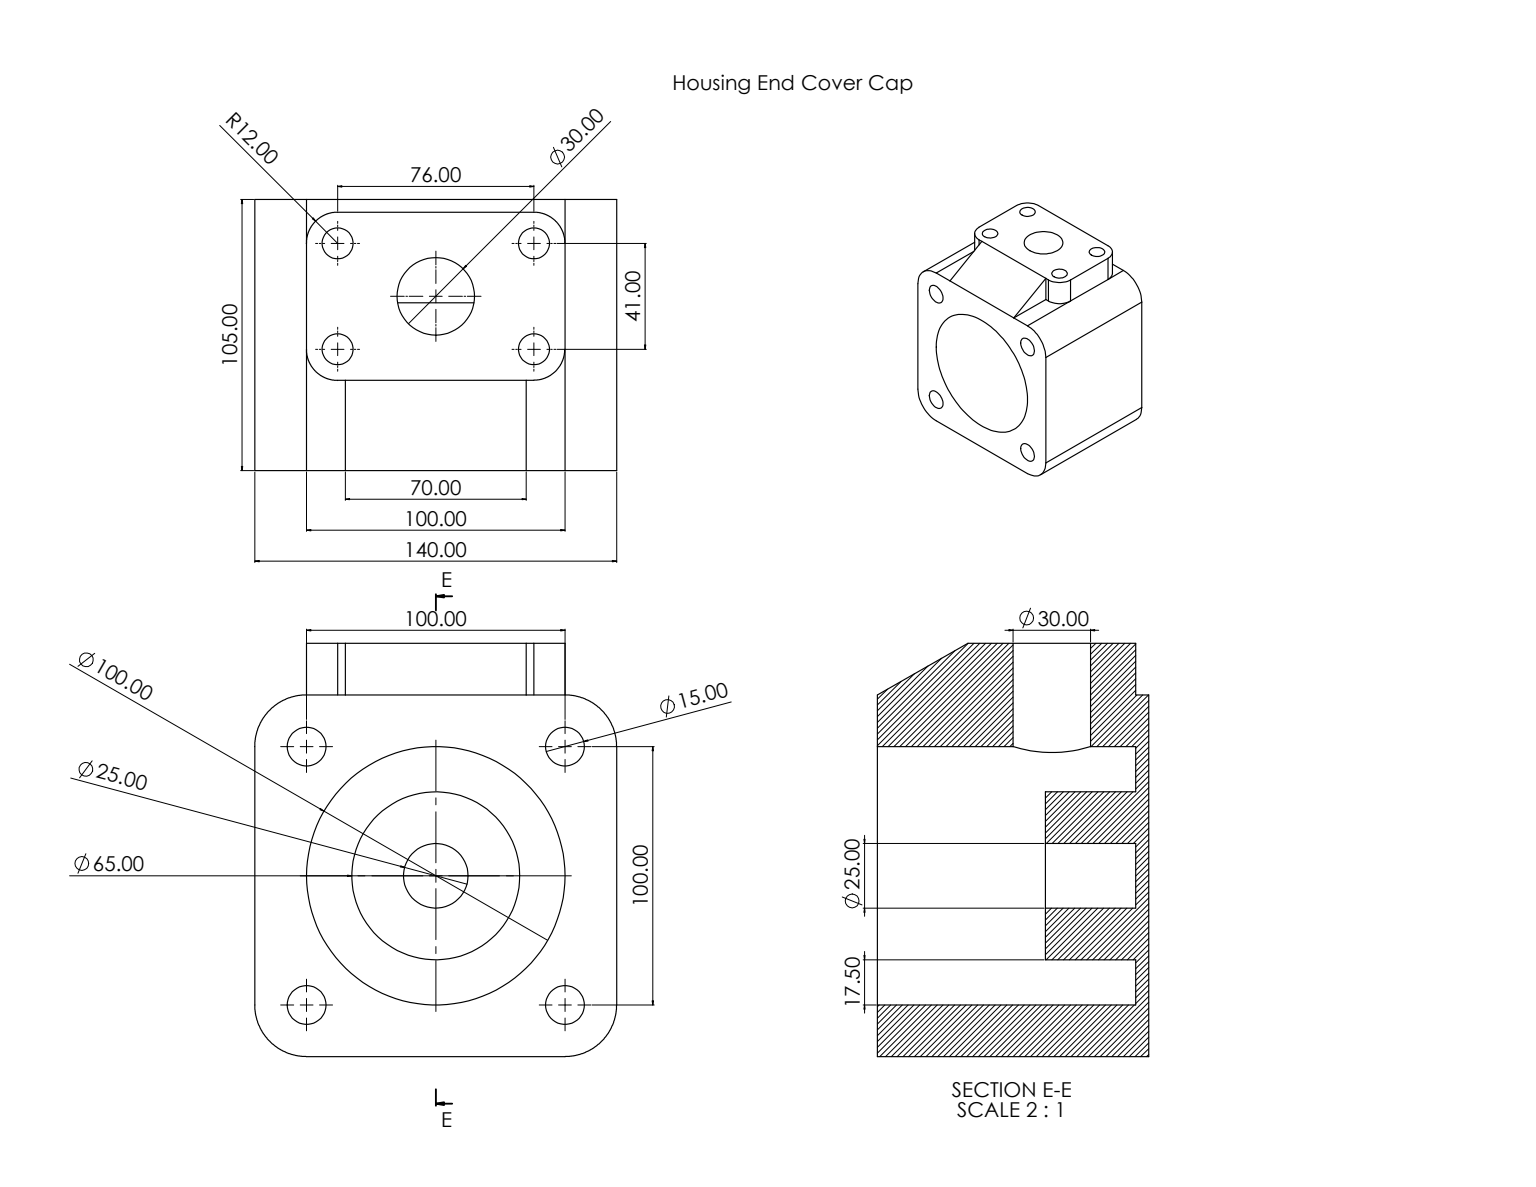
ISO-10303-21;
HEADER;
FILE_DESCRIPTION (('STEP AP214'),
    '1' );
FILE_NAME ('Housing End Cover Cap.step',
    '2026-10-18T20:16:25',
    ( '' ),
    ( '' ),
    'SwSTEP 2.0',
    'SolidWorks 2025',
    '' );
FILE_SCHEMA (( 'AUTOMOTIVE_DESIGN' ));
ENDSEC;

DATA;
#14=CARTESIAN_POINT ( 'NONE',  ( 0.000000000000000000, 0.000000000000000000, 12.49999999999998401 ) ) ;
#20=EDGE_CURVE ( 'NONE', #8430, #1741, #30742, .T. ) ;
#52=VERTEX_POINT ( 'NONE', #10007 ) ;
#62=ADVANCED_FACE ( 'NONE', ( #24650 ), #17167, .F. ) ;
#110=DIRECTION ( 'NONE',  ( 0.000000000000000000, 1.000000000000000000, 0.000000000000000000 ) ) ;
#118=CARTESIAN_POINT ( 'NONE',  ( -12.19297718786180695, 48.49133510641088662, -63.75033992389879245 ) ) ;
#158=DIRECTION ( 'NONE',  ( 1.000000000000000000, 0.000000000000000000, 0.000000000000000000 ) ) ;
#159=VECTOR ( 'NONE', #18850, 1000.000000000000000 ) ;
#182=AXIS2_PLACEMENT_3D ( 'NONE', #29243, #7886, #17394 ) ;
#227=ORIENTED_EDGE ( 'NONE', *, *, #29230, .T. ) ;
#236=ORIENTED_EDGE ( 'NONE', *, *, #10906, .T. ) ;
#272=CARTESIAN_POINT ( 'NONE',  ( -14.80496105867816503, 47.75796600471949205, -57.46067695234416561 ) ) ;
#273=ORIENTED_EDGE ( 'NONE', *, *, #3850, .F. ) ;
#307=ORIENTED_EDGE ( 'NONE', *, *, #24204, .F. ) ;
#319=VECTOR ( 'NONE', #818, 1000.000000000000000 ) ;
#350=DIRECTION ( 'NONE',  ( 1.000000000000000000, -0.000000000000000000, 0.000000000000000000 ) ) ;
#393=PRODUCT_CONTEXT ( 'NONE', #13759, 'mechanical' ) ;
#416=FACE_OUTER_BOUND ( 'NONE', #4200, .T. ) ;
#418=CARTESIAN_POINT ( 'NONE',  ( 37.99999999999999289, 70.00000000000000000, -40.50000000000000711 ) ) ;
#431=EDGE_CURVE ( 'NONE', #20799, #28201, #20243, .T. ) ;
#432=PLANE ( 'NONE',  #5430 ) ;
#444=ORIENTED_EDGE ( 'NONE', *, *, #11235, .F. ) ;
#460=ORIENTED_EDGE ( 'NONE', *, *, #757, .T. ) ;
#480=ADVANCED_FACE ( 'NONE', ( #29613 ), #1231, .F. ) ;
#527=DIRECTION ( 'NONE',  ( -1.000000000000000000, 0.000000000000000000, -0.000000000000000000 ) ) ;
#547=CARTESIAN_POINT ( 'NONE',  ( -42.49999999999998579, -50.00000000000000000, -87.50000000000000000 ) ) ;
#563=CARTESIAN_POINT ( 'NONE',  ( -50.00000000000000000, 50.00000000000000000, 12.49999999999999112 ) ) ;
#572=CARTESIAN_POINT ( 'NONE',  ( -14.87817005273856985, 47.73513060975979982, -56.97185882095643450 ) ) ;
#582=DIRECTION ( 'NONE',  ( -1.000000000000000000, 0.000000000000000000, 0.000000000000000000 ) ) ;
#607=ORIENTED_EDGE ( 'NONE', *, *, #11130, .F. ) ;
#616=ORIENTED_EDGE ( 'NONE', *, *, #19676, .F. ) ;
#635=DIRECTION ( 'NONE',  ( -0.000000000000000000, -1.000000000000000000, -0.000000000000000000 ) ) ;
#656=DIRECTION ( 'NONE',  ( -0.000000000000000000, 1.000000000000000000, -0.000000000000000000 ) ) ;
#660=FACE_OUTER_BOUND ( 'NONE', #25257, .T. ) ;
#661=ORIENTED_EDGE ( 'NONE', *, *, #1590, .T. ) ;
#676=ORIENTED_EDGE ( 'NONE', *, *, #21813, .T. ) ;
#687=CARTESIAN_POINT ( 'NONE',  ( 69.99999999999998579, 50.00000000000000000, 12.49999999999999112 ) ) ;
#689=ORIENTED_EDGE ( 'NONE', *, *, #21785, .F. ) ;
#693=CARTESIAN_POINT ( 'NONE',  ( 35.00000000000000000, 90.00000000000001421, -22.50000000000002487 ) ) ;
#698=AXIS2_PLACEMENT_3D ( 'NONE', #25372, #25055, #15689 ) ;
#715=VECTOR ( 'NONE', #27913, 1000.000000000000000 ) ;
#750=FACE_OUTER_BOUND ( 'NONE', #9838, .T. ) ;
#757=EDGE_CURVE ( 'NONE', #25122, #2838, #4153, .T. ) ;
#806=CARTESIAN_POINT ( 'NONE',  ( 0.000000000000000000, -14.99999999999997158, -40.00000000000000711 ) ) ;
#818=DIRECTION ( 'NONE',  ( 1.000000000000000000, 0.000000000000000000, -1.369518533665900312E-16 ) ) ;
#827=AXIS2_PLACEMENT_3D ( 'NONE', #20012, #14867, #17674 ) ;
#845=DIRECTION ( 'NONE',  ( 1.000000000000000000, 0.000000000000000000, 0.000000000000000000 ) ) ;
#859=CARTESIAN_POINT ( 'NONE',  ( 37.99999999999999289, 90.00000000000001421, -34.50000000000000000 ) ) ;
#878=DIRECTION ( 'NONE',  ( -1.000000000000000000, -0.000000000000000000, -0.000000000000000000 ) ) ;
#892=AXIS2_PLACEMENT_3D ( 'NONE', #11854, #12161, #21660 ) ;
#905=CARTESIAN_POINT ( 'NONE',  ( -37.99999999999999289, 209.2686044187655909, -34.49999999999999289 ) ) ;
#937=AXIS2_PLACEMENT_3D ( 'NONE', #4742, #527, #19100 ) ;
#944=ORIENTED_EDGE ( 'NONE', *, *, #30481, .F. ) ;
#946=VERTEX_POINT ( 'NONE', #18914 ) ;
#988=DIRECTION ( 'NONE',  ( -0.000000000000000000, -0.000000000000000000, -1.000000000000000000 ) ) ;
#991=LINE ( 'NONE', #7551, #25468 ) ;
#1044=DIRECTION ( 'NONE',  ( 0.000000000000000000, 0.000000000000000000, 1.000000000000000000 ) ) ;
#1045=EDGE_LOOP ( 'NONE', ( #21010, #23392 ) ) ;
#1053=CARTESIAN_POINT ( 'NONE',  ( -9.159357180470966142, 49.16077613269642654, -66.91880493524543283 ) ) ;
#1054=( NAMED_UNIT ( * ) PLANE_ANGLE_UNIT ( ) SI_UNIT ( $, .RADIAN. ) );
#1074=LINE ( 'NONE', #29616, #14019 ) ;
#1086=CARTESIAN_POINT ( 'NONE',  ( 49.99999999999998579, -50.00000000000000000, 12.49999999999999112 ) ) ;
#1091=ADVANCED_FACE ( 'NONE', ( #18261 ), #27781, .F. ) ;
#1101=ORIENTED_EDGE ( 'NONE', *, *, #29627, .F. ) ;
#1139=CARTESIAN_POINT ( 'NONE',  ( 13.00588823433103158, 48.28207767711727882, -62.53610571320827916 ) ) ;
#1154=ADVANCED_FACE ( 'NONE', ( #1718 ), #25121, .F. ) ;
#1187=DIRECTION ( 'NONE',  ( 1.000000000000000000, 0.000000000000000000, 0.000000000000000000 ) ) ;
#1191=FACE_OUTER_BOUND ( 'NONE', #19568, .T. ) ;
#1231=PLANE ( 'NONE',  #10135 ) ;
#1241=ORIENTED_EDGE ( 'NONE', *, *, #23033, .F. ) ;
#1248=FACE_OUTER_BOUND ( 'NONE', #28914, .T. ) ;
#1249=AXIS2_PLACEMENT_3D ( 'NONE', #11598, #19076, #21091 ) ;
#1297=CARTESIAN_POINT ( 'NONE',  ( 14.87689969681335178, 47.73552663251712147, -56.98063042392984556 ) ) ;
#1315=ORIENTED_EDGE ( 'NONE', *, *, #26545, .T. ) ;
#1340=ADVANCED_FACE ( 'NONE', ( #14794 ), #21656, .F. ) ;
#1353=ORIENTED_EDGE ( 'NONE', *, *, #8218, .F. ) ;
#1361=( LENGTH_UNIT ( ) NAMED_UNIT ( * ) SI_UNIT ( .MILLI., .METRE. ) );
#1400=ORIENTED_EDGE ( 'NONE', *, *, #2774, .T. ) ;
#1424=AXIS2_PLACEMENT_3D ( 'NONE', #10624, #13592, #15757 ) ;
#1453=VECTOR ( 'NONE', #13826, 1000.000000000000000 ) ;
#1464=CARTESIAN_POINT ( 'NONE',  ( 13.01460760711195519, 48.27982028891777588, -47.47714469611751298 ) ) ;
#1480=ORIENTED_EDGE ( 'NONE', *, *, #24394, .F. ) ;
#1489=EDGE_CURVE ( 'NONE', #8853, #24056, #20553, .T. ) ;
#1494=LINE ( 'NONE', #25341, #4870 ) ;
#1501=ORIENTED_EDGE ( 'NONE', *, *, #17776, .F. ) ;
#1529=EDGE_LOOP ( 'NONE', ( #9098, #1501, #3280, #21052, #26247, #3559 ) ) ;
#1544=DIRECTION ( 'NONE',  ( -0.000000000000000000, -0.000000000000000000, -1.000000000000000000 ) ) ;
#1554=DIRECTION ( 'NONE',  ( 0.000000000000000000, 0.000000000000000000, -1.000000000000000000 ) ) ;
#1570=EDGE_CURVE ( 'NONE', #14635, #28482, #19349, .T. ) ;
#1590=EDGE_CURVE ( 'NONE', #21023, #20390, #27339, .T. ) ;
#1592=EDGE_CURVE ( 'NONE', #21977, #11816, #18995, .T. ) ;
#1606=EDGE_LOOP ( 'NONE', ( #29960, #14559, #1780, #5201 ) ) ;
#1627=DIRECTION ( 'NONE',  ( 0.000000000000000000, 0.000000000000000000, -1.000000000000000000 ) ) ;
#1641=ORIENTED_EDGE ( 'NONE', *, *, #15331, .F. ) ;
#1718=FACE_OUTER_BOUND ( 'NONE', #25812, .T. ) ;
#1728=CARTESIAN_POINT ( 'NONE',  ( -37.99999999999999289, 209.2686044187655909, -75.50000000000000000 ) ) ;
#1741=VERTEX_POINT ( 'NONE', #5257 ) ;
#1751=CARTESIAN_POINT ( 'NONE',  ( 11.90408231459837296, 48.56330485012143328, -64.13958309445501982 ) ) ;
#1755=CARTESIAN_POINT ( 'NONE',  ( -50.00000000000000000, 70.00000000000000000, -92.50000000000000000 ) ) ;
#1766=ADVANCED_FACE ( 'NONE', ( #12444 ), #3221, .F. ) ;
#1767=DIRECTION ( 'NONE',  ( -0.000000000000000000, -0.000000000000000000, -1.000000000000000000 ) ) ;
#1777=DIRECTION ( 'NONE',  ( 0.000000000000000000, 0.000000000000000000, -1.000000000000000000 ) ) ;
#1780=ORIENTED_EDGE ( 'NONE', *, *, #4048, .T. ) ;
#1787=ORIENTED_EDGE ( 'NONE', *, *, #18332, .T. ) ;
#1807=LINE ( 'NONE', #8829, #5442 ) ;
#1827=VERTEX_POINT ( 'NONE', #20372 ) ;
#1845=VERTEX_POINT ( 'NONE', #18039 ) ;
#1858=VECTOR ( 'NONE', #158, 1000.000000000000000 ) ;
#1885=DIRECTION ( 'NONE',  ( -0.000000000000000000, -1.000000000000000000, -0.000000000000000000 ) ) ;
#1891=ORIENTED_EDGE ( 'NONE', *, *, #29175, .F. ) ;
#1897=CARTESIAN_POINT ( 'NONE',  ( 35.00000000000000000, 70.00000000000000000, 12.49999999999999112 ) ) ;
#1936=EDGE_CURVE ( 'NONE', #1827, #23754, #10864, .T. ) ;
#1960=DIRECTION ( 'NONE',  ( -1.000000000000000000, 0.000000000000000000, 0.000000000000000000 ) ) ;
#1965=EDGE_CURVE ( 'NONE', #6185, #27407, #6927, .T. ) ;
#1993=CYLINDRICAL_SURFACE ( 'NONE', #11539, 7.500000000000013323 ) ;
#2043=FACE_OUTER_BOUND ( 'NONE', #24533, .T. ) ;
#2100=ADVANCED_FACE ( 'NONE', ( #25824 ), #20824, .F. ) ;
#2126=VECTOR ( 'NONE', #2316, 1000.000000000000000 ) ;
#2140=FACE_OUTER_BOUND ( 'NONE', #17021, .T. ) ;
#2184=CARTESIAN_POINT ( 'NONE',  ( 49.99999999999998579, -50.00000000000000000, 12.49999999999998401 ) ) ;
#2192=EDGE_LOOP ( 'NONE', ( #1641, #28752 ) ) ;
#2197=DIRECTION ( 'NONE',  ( 0.000000000000000000, 1.000000000000000000, 0.000000000000000000 ) ) ;
#2233=VERTEX_POINT ( 'NONE', #27703 ) ;
#2249=AXIS2_PLACEMENT_3D ( 'NONE', #8441, #17784, #27145 ) ;
#2267=ORIENTED_EDGE ( 'NONE', *, *, #11841, .F. ) ;
#2275=ADVANCED_FACE ( 'NONE', ( #22124, #27555, #25049, #17464, #14800, #750 ), #2967, .T. ) ;
#2282=DIRECTION ( 'NONE',  ( 0.000000000000000000, 0.000000000000000000, 1.000000000000000000 ) ) ;
#2295=CARTESIAN_POINT ( 'NONE',  ( -50.00000000000000000, 50.00000000000000000, -92.50000000000000000 ) ) ;
#2316=DIRECTION ( 'NONE',  ( 0.000000000000000000, 0.000000000000000000, -1.000000000000000000 ) ) ;
#2320=EDGE_CURVE ( 'NONE', #6658, #18599, #1807, .T. ) ;
#2327=CYLINDRICAL_SURFACE ( 'NONE', #892, 50.00000000000000000 ) ;
#2349=CYLINDRICAL_SURFACE ( 'NONE', #18326, 20.00000000000000355 ) ;
#2357=ORIENTED_EDGE ( 'NONE', *, *, #7891, .F. ) ;
#2361=CARTESIAN_POINT ( 'NONE',  ( 0.9970077338578161585, 49.99999999999997158, -40.00000000000000000 ) ) ;
#2378=EDGE_CURVE ( 'NONE', #27015, #15437, #25366, .T. ) ;
#2444=VERTEX_POINT ( 'NONE', #18011 ) ;
#2466=CARTESIAN_POINT ( 'NONE',  ( -13.66184973646045542, 48.09774150583283614, -61.21269189572690550 ) ) ;
#2476=LINE ( 'NONE', #28981, #6020 ) ;
#2552=LINE ( 'NONE', #7843, #9206 ) ;
#2573=FACE_OUTER_BOUND ( 'NONE', #1606, .T. ) ;
#2606=CARTESIAN_POINT ( 'NONE',  ( 37.99999999999999289, 209.2686044187655909, -75.50000000000001421 ) ) ;
#2607=DIRECTION ( 'NONE',  ( -1.000000000000000000, 0.000000000000000000, 0.000000000000000000 ) ) ;
#2610=ORIENTED_EDGE ( 'NONE', *, *, #5389, .T. ) ;
#2616=CARTESIAN_POINT ( 'NONE',  ( -1.976776171439267760, 49.97021316353860954, -40.09845666013538334 ) ) ;
#2625=ORIENTED_EDGE ( 'NONE', *, *, #17830, .F. ) ;
#2629=EDGE_LOOP ( 'NONE', ( #21905, #1400, #4052, #5248 ) ) ;
#2635=AXIS2_PLACEMENT_3D ( 'NONE', #25004, #29387, #3644 ) ;
#2641=DIRECTION ( 'NONE',  ( -0.000000000000000000, -1.000000000000000000, -0.000000000000000000 ) ) ;
#2642=CARTESIAN_POINT ( 'NONE',  ( 37.99999999999999289, 90.00000000000001421, -69.50000000000000000 ) ) ;
#2647=AXIS2_PLACEMENT_3D ( 'NONE', #20182, #29706, #3977 ) ;
#2650=DIRECTION ( 'NONE',  ( -0.000000000000000000, -0.000000000000000000, -1.000000000000000000 ) ) ;
#2664=CYLINDRICAL_SURFACE ( 'NONE', #18902, 32.50000000000000000 ) ;
#2676=ORIENTED_EDGE ( 'NONE', *, *, #19295, .F. ) ;
#2684=AXIS2_PLACEMENT_3D ( 'NONE', #4117, #13647, #4419 ) ;
#2685=CARTESIAN_POINT ( 'NONE',  ( 49.99999999999998579, 50.00000000000000000, 52.07879600563550326 ) ) ;
#2688=AXIS2_PLACEMENT_3D ( 'NONE', #14981, #7816, #8133 ) ;
#2725=ORIENTED_EDGE ( 'NONE', *, *, #6905, .F. ) ;
#2745=ADVANCED_FACE ( 'NONE', ( #15301 ), #3467, .F. ) ;
#2772=VERTEX_POINT ( 'NONE', #18122 ) ;
#2774=EDGE_CURVE ( 'NONE', #15471, #8734, #18703, .T. ) ;
#2775=CARTESIAN_POINT ( 'NONE',  ( -9.910680102653831369, 49.01306433446774946, -66.30206827149085314 ) ) ;
#2792=CIRCLE ( 'NONE', #4278, 50.00000000000000000 ) ;
#2835=CIRCLE ( 'NONE', #10815, 50.00000000000000000 ) ;
#2838=VERTEX_POINT ( 'NONE', #10894 ) ;
#2853=AXIS2_PLACEMENT_3D ( 'NONE', #12741, #29431, #29274 ) ;
#2855=LINE ( 'NONE', #5194, #24404 ) ;
#2859=CARTESIAN_POINT ( 'NONE',  ( -37.99999999999999289, 70.00000000000000000, -22.50000000000001421 ) ) ;
#2861=EDGE_LOOP ( 'NONE', ( #28394, #10437, #4508, #19072 ) ) ;
#2873=CIRCLE ( 'NONE', #22303, 7.500000000000013323 ) ;
#2877=CARTESIAN_POINT ( 'NONE',  ( -42.49999999999998579, 50.00000000000000000, 12.49999999999999112 ) ) ;
#2888=EDGE_LOOP ( 'NONE', ( #25502, #20285, #18915 ) ) ;
#2908=CYLINDRICAL_SURFACE ( 'NONE', #25297, 7.500000000000013323 ) ;
#2921=DIRECTION ( 'NONE',  ( -0.000000000000000000, -0.000000000000000000, 1.000000000000000000 ) ) ;
#2935=EDGE_LOOP ( 'NONE', ( #18951, #15081, #30148, #25140 ) ) ;
#2937=CARTESIAN_POINT ( 'NONE',  ( -14.90305376050273267, 47.72777027336211120, -53.03111353900148117 ) ) ;
#2967=PLANE ( 'NONE',  #23352 ) ;
#3004=DIRECTION ( 'NONE',  ( -0.000000000000000000, -0.000000000000000000, 1.000000000000000000 ) ) ;
#3009=LINE ( 'NONE', #21872, #30467 ) ;
#3011=DIRECTION ( 'NONE',  ( -0.000000000000000000, -0.000000000000000000, -1.000000000000000000 ) ) ;
#3023=DIRECTION ( 'NONE',  ( 0.000000000000000000, 0.000000000000000000, -1.000000000000000000 ) ) ;
#3033=DIRECTION ( 'NONE',  ( 1.000000000000000000, 0.000000000000000000, -0.000000000000000000 ) ) ;
#3041=ORIENTED_EDGE ( 'NONE', *, *, #21813, .F. ) ;
#3053=DIRECTION ( 'NONE',  ( 0.000000000000000000, 0.000000000000000000, -1.000000000000000000 ) ) ;
#3055=ORIENTED_EDGE ( 'NONE', *, *, #15547, .T. ) ;
#3067=CARTESIAN_POINT ( 'NONE',  ( -37.99999999999999289, 209.2686044187655909, -22.50000000000000711 ) ) ;
#3073=DIRECTION ( 'NONE',  ( 0.000000000000000000, 0.000000000000000000, -1.000000000000000000 ) ) ;
#3080=CARTESIAN_POINT ( 'NONE',  ( -14.23021073309091733, 47.93387744827222718, -59.84518500609045333 ) ) ;
#3092=DIRECTION ( 'NONE',  ( 0.000000000000000000, 0.000000000000000000, -1.000000000000000000 ) ) ;
#3124=ADVANCED_FACE ( 'NONE', ( #1191 ), #17710, .F. ) ;
#3134=ADVANCED_FACE ( 'NONE', ( #22686 ), #27231, .F. ) ;
#3175=MANIFOLD_SOLID_BREP ( 'Boss-Extrude22', #18321 ) ;
#3182=DIRECTION ( 'NONE',  ( 0.000000000000000000, -0.000000000000000000, -1.000000000000000000 ) ) ;
#3204=CARTESIAN_POINT ( 'NONE',  ( 49.99999999999998579, -50.00000000000000000, 52.07879600563550326 ) ) ;
#3214=( NAMED_UNIT ( * ) SI_UNIT ( $, .STERADIAN. ) SOLID_ANGLE_UNIT ( ) );
#3221=CYLINDRICAL_SURFACE ( 'NONE', #20837, 12.50000000000000000 ) ;
#3251=DIRECTION ( 'NONE',  ( 0.000000000000000000, 0.000000000000000000, 1.000000000000000000 ) ) ;
#3266=EDGE_LOOP ( 'NONE', ( #24974, #25472 ) ) ;
#3280=ORIENTED_EDGE ( 'NONE', *, *, #9923, .F. ) ;
#3287=AXIS2_PLACEMENT_3D ( 'NONE', #9817, #19330, #3251 ) ;
#3301=CARTESIAN_POINT ( 'NONE',  ( 37.99999999999999289, 90.00000000000001421, -34.50000000000000000 ) ) ;
#3306=AXIS2_PLACEMENT_3D ( 'NONE', #14798, #24620, #7488 ) ;
#3320=CARTESIAN_POINT ( 'NONE',  ( 42.49999999999998579, -50.00000000000000000, -87.50000000000000000 ) ) ;
#3353=AXIS2_PLACEMENT_3D ( 'NONE', #25352, #13355, #20660 ) ;
#3388=CARTESIAN_POINT ( 'NONE',  ( -6.651921343684833232, 49.55749932660967971, -68.45349145285689474 ) ) ;
#3413=CARTESIAN_POINT ( 'NONE',  ( -70.00000000000000000, -50.00000000000000000, 12.49999999999999112 ) ) ;
#3428=CARTESIAN_POINT ( 'NONE',  ( -37.99999999999999289, 90.00000000000001421, -69.49999999999998579 ) ) ;
#3467=PLANE ( 'NONE',  #17748 ) ;
#3500=EDGE_CURVE ( 'NONE', #10117, #26490, #26497, .T. ) ;
#3538=CARTESIAN_POINT ( 'NONE',  ( 49.99999999999998579, 90.00000000000001421, -75.50000000000001421 ) ) ;
#3547=CARTESIAN_POINT ( 'NONE',  ( -35.00000000000000000, 70.00000000000000000, -22.50000000000003908 ) ) ;
#3550=ORIENTED_EDGE ( 'NONE', *, *, #30763, .T. ) ;
#3559=ORIENTED_EDGE ( 'NONE', *, *, #3500, .F. ) ;
#3583=DIRECTION ( 'NONE',  ( 0.000000000000000000, -0.000000000000000000, -1.000000000000000000 ) ) ;
#3586=VECTOR ( 'NONE', #6850, 1000.000000000000000 ) ;
#3589=LINE ( 'NONE', #5627, #4488 ) ;
#3644=DIRECTION ( 'NONE',  ( -1.000000000000000000, 0.000000000000000000, 1.369518533665900065E-16 ) ) ;
#3678=CIRCLE ( 'NONE', #4661, 20.00000000000000000 ) ;
#3679=EDGE_CURVE ( 'NONE', #11709, #22434, #4291, .T. ) ;
#3690=DIRECTION ( 'NONE',  ( -1.000000000000000000, -0.000000000000000000, -0.000000000000000000 ) ) ;
#3704=EDGE_CURVE ( 'NONE', #8734, #15471, #6786, .T. ) ;
#3737=ORIENTED_EDGE ( 'NONE', *, *, #11495, .T. ) ;
#3767=EDGE_CURVE ( 'NONE', #30269, #15581, #4172, .T. ) ;
#3770=EDGE_LOOP ( 'NONE', ( #6397, #9480, #13738, #18719 ) ) ;
#3772=CARTESIAN_POINT ( 'NONE',  ( -35.00000000000000000, 90.00000000000001421, -22.50000000000002487 ) ) ;
#3792=CARTESIAN_POINT ( 'NONE',  ( 11.28349294625599519, 48.71123628743529821, -64.89555161802378791 ) ) ;
#3801=DIRECTION ( 'NONE',  ( -1.000000000000000000, 0.000000000000000000, -0.000000000000000000 ) ) ;
#3803=VECTOR ( 'NONE', #4068, 1000.000000000000000 ) ;
#3814=EDGE_LOOP ( 'NONE', ( #26252, #27150 ) ) ;
#3839=AXIS2_PLACEMENT_3D ( 'NONE', #29893, #20367, #5557 ) ;
#3841=ADVANCED_FACE ( 'NONE', ( #416 ), #12441, .F. ) ;
#3850=EDGE_CURVE ( 'NONE', #27558, #2772, #26201, .T. ) ;
#3877=EDGE_CURVE ( 'NONE', #26519, #8036, #4779, .T. ) ;
#3885=DIRECTION ( 'NONE',  ( 0.000000000000000000, 0.000000000000000000, -1.000000000000000000 ) ) ;
#3888=CIRCLE ( 'NONE', #12866, 11.99999999999998934 ) ;
#3897=DIRECTION ( 'NONE',  ( -1.000000000000000000, 0.000000000000000000, 0.000000000000000000 ) ) ;
#3934=LINE ( 'NONE', #3772, #26256 ) ;
#3939=CARTESIAN_POINT ( 'NONE',  ( -37.99999999999999289, 90.00000000000001421, -75.50000000000000000 ) ) ;
#3957=CARTESIAN_POINT ( 'NONE',  ( 10.95142783224707550, 48.78720750482332846, -65.26185492559442025 ) ) ;
#3976=VERTEX_POINT ( 'NONE', #4945 ) ;
#3977=DIRECTION ( 'NONE',  ( 0.000000000000000000, -0.000000000000000000, -1.000000000000000000 ) ) ;
#3985=LINE ( 'NONE', #13508, #29816 ) ;
#4016=APPLICATION_CONTEXT ( 'automotive_design' ) ;
#4048=EDGE_CURVE ( 'NONE', #27691, #1845, #12903, .T. ) ;
#4052=ORIENTED_EDGE ( 'NONE', *, *, #22560, .T. ) ;
#4059=LINE ( 'NONE', #20579, #17067 ) ;
#4068=DIRECTION ( 'NONE',  ( -0.000000000000000000, -1.000000000000000000, -0.000000000000000000 ) ) ;
#4078=DIRECTION ( 'NONE',  ( -1.000000000000000000, 0.000000000000000000, 0.000000000000000000 ) ) ;
#4088=DIRECTION ( 'NONE',  ( -0.000000000000000000, -1.000000000000000000, -0.000000000000000000 ) ) ;
#4090=DIRECTION ( 'NONE',  ( 1.000000000000000000, 0.000000000000000000, 0.000000000000000000 ) ) ;
#4094=ORIENTED_EDGE ( 'NONE', *, *, #2774, .F. ) ;
#4103=VERTEX_POINT ( 'NONE', #29726 ) ;
#4117=CARTESIAN_POINT ( 'NONE',  ( -37.99999999999999289, 209.2686044187655909, -22.50000000000001421 ) ) ;
#4153=CIRCLE ( 'NONE', #18608, 6.000000000000005329 ) ;
#4156=CIRCLE ( 'NONE', #21578, 20.00000000000000355 ) ;
#4172=LINE ( 'NONE', #29112, #30193 ) ;
#4177=ORIENTED_EDGE ( 'NONE', *, *, #7257, .F. ) ;
#4193=ORIENTED_EDGE ( 'NONE', *, *, #28094, .F. ) ;
#4200=EDGE_LOOP ( 'NONE', ( #22486, #236, #24354, #13821 ) ) ;
#4205=DIRECTION ( 'NONE',  ( 0.000000000000000000, 1.000000000000000000, 6.938893903907227392E-16 ) ) ;
#4217=PLANE ( 'NONE',  #27251 ) ;
#4229=LINE ( 'NONE', #23548, #16439 ) ;
#4239=CARTESIAN_POINT ( 'NONE',  ( 5.317332916452814473, 49.71854057255719539, -40.96554122676177201 ) ) ;
#4258=CARTESIAN_POINT ( 'NONE',  ( 49.99999999999998579, 50.00000000000000000, 12.49999999999999112 ) ) ;
#4268=FACE_OUTER_BOUND ( 'NONE', #21376, .T. ) ;
#4278=AXIS2_PLACEMENT_3D ( 'NONE', #19953, #15105, #29472 ) ;
#4291=CIRCLE ( 'NONE', #20236, 32.50000000000000000 ) ;
#4292=ORIENTED_EDGE ( 'NONE', *, *, #17776, .T. ) ;
#4330=CIRCLE ( 'NONE', #21760, 6.000000000000005329 ) ;
#4347=AXIS2_PLACEMENT_3D ( 'NONE', #15874, #16484, #30657 ) ;
#4352=ORIENTED_EDGE ( 'NONE', *, *, #27680, .T. ) ;
#4372=FACE_OUTER_BOUND ( 'NONE', #27020, .T. ) ;
#4379=AXIS2_PLACEMENT_3D ( 'NONE', #26165, #16192, #11528 ) ;
#4395=ADVANCED_FACE ( 'NONE', ( #25157 ), #17381, .F. ) ;
#4419=DIRECTION ( 'NONE',  ( -1.000000000000000000, 0.000000000000000000, 1.369518533665900065E-16 ) ) ;
#4488=VECTOR ( 'NONE', #29638, 1000.000000000000000 ) ;
#4490=DIRECTION ( 'NONE',  ( 0.000000000000000000, 0.000000000000000000, -1.000000000000000000 ) ) ;
#4508=ORIENTED_EDGE ( 'NONE', *, *, #27657, .T. ) ;
#4538=LINE ( 'NONE', #5308, #1858 ) ;
#4559=ORIENTED_EDGE ( 'NONE', *, *, #5602, .T. ) ;
#4569=DIRECTION ( 'NONE',  ( -1.000000000000000000, 0.000000000000000000, 0.000000000000000000 ) ) ;
#4578=EDGE_LOOP ( 'NONE', ( #24122, #21961 ) ) ;
#4580=VECTOR ( 'NONE', #22281, 1000.000000000000000 ) ;
#4603=DIRECTION ( 'NONE',  ( 0.000000000000000000, 1.000000000000000000, 0.000000000000000000 ) ) ;
#4609=CARTESIAN_POINT ( 'NONE',  ( -37.99999999999999289, 209.2686044187655909, -81.50000000000000000 ) ) ;
#4635=FACE_BOUND ( 'NONE', #30165, .T. ) ;
#4649=VERTEX_POINT ( 'NONE', #26397 ) ;
#4661=AXIS2_PLACEMENT_3D ( 'NONE', #2184, #28861, #23999 ) ;
#4671=ORIENTED_EDGE ( 'NONE', *, *, #26545, .F. ) ;
#4690=DIRECTION ( 'NONE',  ( 0.000000000000000000, 0.000000000000000000, -1.000000000000000000 ) ) ;
#4698=CARTESIAN_POINT ( 'NONE',  ( 1.868132521858655084E-15, 50.00000000000000000, -40.00000000000000711 ) ) ;
#4726=ORIENTED_EDGE ( 'NONE', *, *, #20656, .T. ) ;
#4727=CIRCLE ( 'NONE', #23636, 32.50000000000000000 ) ;
#4742=CARTESIAN_POINT ( 'NONE',  ( 69.99999999999998579, 70.00000000000000000, -92.50000000000000000 ) ) ;
#4752=ORIENTED_EDGE ( 'NONE', *, *, #5216, .F. ) ;
#4779=LINE ( 'NONE', #3067, #23204 ) ;
#4805=ORIENTED_EDGE ( 'NONE', *, *, #3767, .F. ) ;
#4810=AXIS2_PLACEMENT_3D ( 'NONE', #5511, #20009, #3023 ) ;
#4842=CARTESIAN_POINT ( 'NONE',  ( -50.00000000000000000, -50.00000000000000000, -87.50000000000000000 ) ) ;
#4870=VECTOR ( 'NONE', #29883, 1000.000000000000000 ) ;
#4873=AXIS2_PLACEMENT_3D ( 'NONE', #30449, #16414, #28120 ) ;
#4876=EDGE_LOOP ( 'NONE', ( #30060, #10543, #29266, #29368 ) ) ;
#4943=PRODUCT ( 'Housing End Cover Cap', 'Housing End Cover Cap', '', ( #393 ) ) ;
#4945=CARTESIAN_POINT ( 'NONE',  ( 50.00000000000000000, 6.123233995736766085E-15, 12.49999999999998401 ) ) ;
#4957=CARTESIAN_POINT ( 'NONE',  ( -14.99954637771879540, 47.69710272843848742, -54.00831070145920165 ) ) ;
#4994=AXIS2_PLACEMENT_3D ( 'NONE', #5814, #27033, #22484 ) ;
#5006=DIRECTION ( 'NONE',  ( -1.000000000000000000, 0.000000000000000000, 0.000000000000000000 ) ) ;
#5028=ADVANCED_FACE ( 'NONE', ( #24731 ), #7753, .F. ) ;
#5062=EDGE_CURVE ( 'NONE', #11207, #18139, #5863, .T. ) ;
#5125=EDGE_LOOP ( 'NONE', ( #29214, #24225, #27771, #17870 ) ) ;
#5129=DIRECTION ( 'NONE',  ( -1.000000000000000000, 0.000000000000000000, 0.000000000000000000 ) ) ;
#5130=CIRCLE ( 'NONE', #22562, 7.500000000000000000 ) ;
#5179=CARTESIAN_POINT ( 'NONE',  ( -70.00000000000000000, -50.00000000000000000, -92.50000000000000000 ) ) ;
#5182=AXIS2_PLACEMENT_3D ( 'NONE', #19514, #24649, #22310 ) ;
#5194=CARTESIAN_POINT ( 'NONE',  ( 38.00000000000000711, 209.2686044187655909, -87.50000000000000000 ) ) ;
#5201=ORIENTED_EDGE ( 'NONE', *, *, #28277, .F. ) ;
#5216=EDGE_CURVE ( 'NONE', #20799, #22863, #20516, .T. ) ;
#5228=VECTOR ( 'NONE', #22063, 1000.000000000000000 ) ;
#5231=DIRECTION ( 'NONE',  ( 0.000000000000000000, 1.000000000000000000, 0.000000000000000000 ) ) ;
#5232=EDGE_LOOP ( 'NONE', ( #2676, #23041 ) ) ;
#5248=ORIENTED_EDGE ( 'NONE', *, *, #18916, .F. ) ;
#5257=CARTESIAN_POINT ( 'NONE',  ( -50.00000000000000000, -70.00000000000000000, 12.49999999999999112 ) ) ;
#5276=EDGE_CURVE ( 'NONE', #20799, #23754, #17713, .T. ) ;
#5308=CARTESIAN_POINT ( 'NONE',  ( -70.00000000000000000, 70.00000000000000000, -92.50000000000000000 ) ) ;
#5351=CARTESIAN_POINT ( 'NONE',  ( 32.50000000000000000, 3.980102097228898626E-15, -87.50000000000000000 ) ) ;
#5365=CARTESIAN_POINT ( 'NONE',  ( -49.99999999999998579, 70.00000000000000000, -75.50000000000002842 ) ) ;
#5370=ORIENTED_EDGE ( 'NONE', *, *, #1570, .F. ) ;
#5389=EDGE_CURVE ( 'NONE', #6549, #28201, #6849, .T. ) ;
#5391=ADVANCED_FACE ( 'NONE', ( #6780 ), #18959, .F. ) ;
#5396=VECTOR ( 'NONE', #27361, 1000.000000000000000 ) ;
#5412=DIRECTION ( 'NONE',  ( 0.000000000000000000, 0.000000000000000000, -1.000000000000000000 ) ) ;
#5427=CARTESIAN_POINT ( 'NONE',  ( -6.672226544319371122, 49.56122815818398664, -41.52977849429709067 ) ) ;
#5429=ORIENTED_EDGE ( 'NONE', *, *, #18916, .T. ) ;
#5430=AXIS2_PLACEMENT_3D ( 'NONE', #21476, #23969, #12600 ) ;
#5442=VECTOR ( 'NONE', #21116, 1000.000000000000000 ) ;
#5467=CARTESIAN_POINT ( 'NONE',  ( -35.00000000000000000, 70.00000000000000000, 12.49999999999999112 ) ) ;
#5498=CARTESIAN_POINT ( 'NONE',  ( 0.000000000000000000, 0.000000000000000000, 12.49999999999999112 ) ) ;
#5499=LINE ( 'NONE', #806, #9917 ) ;
#5502=DIRECTION ( 'NONE',  ( -1.000000000000000000, 0.000000000000000000, 0.000000000000000000 ) ) ;
#5511=CARTESIAN_POINT ( 'NONE',  ( -37.99999999999999289, 70.00000000000000000, -34.49999999999999289 ) ) ;
#5514=DIRECTION ( 'NONE',  ( -0.000000000000000000, -0.000000000000000000, 1.000000000000000000 ) ) ;
#5543=DIRECTION ( 'NONE',  ( 0.000000000000000000, 0.000000000000000000, -1.000000000000000000 ) ) ;
#5544=DIRECTION ( 'NONE',  ( -1.000000000000000000, 0.000000000000000000, 0.000000000000000000 ) ) ;
#5546=EDGE_LOOP ( 'NONE', ( #24679, #8107 ) ) ;
#5553=ORIENTED_EDGE ( 'NONE', *, *, #12219, .F. ) ;
#5557=DIRECTION ( 'NONE',  ( -1.000000000000000000, 0.000000000000000000, 0.000000000000000000 ) ) ;
#5558=EDGE_CURVE ( 'NONE', #29647, #18139, #22368, .T. ) ;
#5562=DIRECTION ( 'NONE',  ( -1.000000000000000000, 0.000000000000000000, 0.000000000000000000 ) ) ;
#5576=CARTESIAN_POINT ( 'NONE',  ( -4.851473655640472948, 49.77239851816440108, -69.22750204485392089 ) ) ;
#5584=ORIENTED_EDGE ( 'NONE', *, *, #16213, .T. ) ;
#5602=EDGE_CURVE ( 'NONE', #15417, #30269, #28429, .T. ) ;
#5625=CARTESIAN_POINT ( 'NONE',  ( 69.99999999999998579, 70.00000000000000000, -92.50000000000000000 ) ) ;
#5626=FACE_OUTER_BOUND ( 'NONE', #15609, .T. ) ;
#5627=CARTESIAN_POINT ( 'NONE',  ( -50.00000000000000000, -70.00000000000000000, -92.50000000000000000 ) ) ;
#5638=FACE_OUTER_BOUND ( 'NONE', #5125, .T. ) ;
#5663=DIRECTION ( 'NONE',  ( 1.000000000000000000, 0.000000000000000000, -1.369518533665900065E-16 ) ) ;
#5688=DIRECTION ( 'NONE',  ( 0.000000000000000000, -0.000000000000000000, 1.000000000000000000 ) ) ;
#5733=DIRECTION ( 'NONE',  ( -0.000000000000000000, -1.000000000000000000, -0.000000000000000000 ) ) ;
#5764=EDGE_CURVE ( 'NONE', #10221, #20799, #24035, .T. ) ;
#5776=DIRECTION ( 'NONE',  ( 0.000000000000000000, 0.000000000000000000, -1.000000000000000000 ) ) ;
#5814=CARTESIAN_POINT ( 'NONE',  ( 0.000000000000000000, 0.000000000000000000, -87.50000000000000000 ) ) ;
#5815=ORIENTED_EDGE ( 'NONE', *, *, #24003, .F. ) ;
#5817=CYLINDRICAL_SURFACE ( 'NONE', #7460, 15.00000000000000000 ) ;
#5822=CARTESIAN_POINT ( 'NONE',  ( 14.22989400835912832, 47.93398237600714396, -59.84665844486981001 ) ) ;
#5852=ORIENTED_EDGE ( 'NONE', *, *, #7671, .T. ) ;
#5863=CIRCLE ( 'NONE', #25301, 7.500000000000013323 ) ;
#5873=CARTESIAN_POINT ( 'NONE',  ( -70.00000000000000000, 70.00000000000000000, 12.49999999999999112 ) ) ;
#5894=ORIENTED_EDGE ( 'NONE', *, *, #14922, .T. ) ;
#5897=DIRECTION ( 'NONE',  ( 0.000000000000000000, 0.000000000000000000, -1.000000000000000000 ) ) ;
#5905=AXIS2_PLACEMENT_3D ( 'NONE', #21469, #110, #9630 ) ;
#5915=CARTESIAN_POINT ( 'NONE',  ( 35.00000000000000000, 90.00000000000001421, -22.50000000000002487 ) ) ;
#5947=CARTESIAN_POINT ( 'NONE',  ( 35.00000000000000000, 70.00000000000000000, -22.50000000000003908 ) ) ;
#5958=CARTESIAN_POINT ( 'NONE',  ( 37.99999999999999289, 70.00000000000000000, -69.50000000000000000 ) ) ;
#5969=ORIENTED_EDGE ( 'NONE', *, *, #20809, .F. ) ;
#5979=CARTESIAN_POINT ( 'NONE',  ( 2.454608198648450479, 49.94209336002347044, -69.80612517421458563 ) ) ;
#6020=VECTOR ( 'NONE', #26334, 1000.000000000000000 ) ;
#6040=CARTESIAN_POINT ( 'NONE',  ( -37.99999999999999289, 209.2686044187655909, -69.49999999999998579 ) ) ;
#6101=DIRECTION ( 'NONE',  ( -1.000000000000000000, 0.000000000000000000, -0.000000000000000000 ) ) ;
#6124=CARTESIAN_POINT ( 'NONE',  ( 11.91715319254153371, 48.56235700707689062, -45.83731355574434474 ) ) ;
#6156=ORIENTED_EDGE ( 'NONE', *, *, #23869, .T. ) ;
#6185=VERTEX_POINT ( 'NONE', #29121 ) ;
#6205=CARTESIAN_POINT ( 'NONE',  ( 37.99999999999999289, 209.2686044187655909, -34.50000000000000000 ) ) ;
#6206=ORIENTED_EDGE ( 'NONE', *, *, #16258, .T. ) ;
#6226=DIRECTION ( 'NONE',  ( -0.000000000000000000, -1.000000000000000000, -0.000000000000000000 ) ) ;
#6248=CARTESIAN_POINT ( 'NONE',  ( 35.00000000000000000, 0.000000000000000000, 0.000000000000000000 ) ) ;
#6272=CARTESIAN_POINT ( 'NONE',  ( 0.000000000000000000, -14.99999999999997158, -55.00000000000000711 ) ) ;
#6273=CIRCLE ( 'NONE', #3287, 15.00000000000000000 ) ;
#6287=DIRECTION ( 'NONE',  ( -0.000000000000000000, -1.000000000000000000, -0.000000000000000000 ) ) ;
#6290=AXIS2_PLACEMENT_3D ( 'NONE', #11662, #23810, #18997 ) ;
#6317=VECTOR ( 'NONE', #8954, 1000.000000000000000 ) ;
#6362=FACE_OUTER_BOUND ( 'NONE', #14584, .T. ) ;
#6397=ORIENTED_EDGE ( 'NONE', *, *, #9642, .T. ) ;
#6400=ORIENTED_EDGE ( 'NONE', *, *, #12419, .T. ) ;
#6412=CARTESIAN_POINT ( 'NONE',  ( 37.99999999999999289, 209.2686044187655909, -75.50000000000001421 ) ) ;
#6418=DIRECTION ( 'NONE',  ( 0.000000000000000000, -0.4961389383568337030, 0.8682431421244592995 ) ) ;
#6423=VECTOR ( 'NONE', #26742, 1000.000000000000000 ) ;
#6443=CARTESIAN_POINT ( 'NONE',  ( 7.522556813806144937, 49.43282481825458774, -67.98671092651753156 ) ) ;
#6447=VECTOR ( 'NONE', #25194, 1000.000000000000000 ) ;
#6464=PLANE ( 'NONE',  #2684 ) ;
#6469=DIRECTION ( 'NONE',  ( -1.000000000000000000, 0.000000000000000000, 0.000000000000000000 ) ) ;
#6490=AXIS2_PLACEMENT_3D ( 'NONE', #4842, #4690, #11877 ) ;
#6494=EDGE_CURVE ( 'NONE', #12057, #7501, #21061, .T. ) ;
#6515=DIRECTION ( 'NONE',  ( 0.000000000000000000, -0.000000000000000000, -1.000000000000000000 ) ) ;
#6533=ADVANCED_FACE ( 'NONE', ( #17386 ), #21742, .T. ) ;
#6538=CARTESIAN_POINT ( 'NONE',  ( 37.99999999999999289, 70.00000000000000000, -34.50000000000000000 ) ) ;
#6549=VERTEX_POINT ( 'NONE', #687 ) ;
#6626=CYLINDRICAL_SURFACE ( 'NONE', #3353, 15.00000000000000000 ) ;
#6635=DIRECTION ( 'NONE',  ( 0.000000000000000000, 0.000000000000000000, 1.000000000000000000 ) ) ;
#6649=ORIENTED_EDGE ( 'NONE', *, *, #15667, .T. ) ;
#6658=VERTEX_POINT ( 'NONE', #24085 ) ;
#6727=ORIENTED_EDGE ( 'NONE', *, *, #29150, .F. ) ;
#6780=FACE_OUTER_BOUND ( 'NONE', #2629, .T. ) ;
#6786=CIRCLE ( 'NONE', #10283, 6.000000000000005329 ) ;
#6792=LINE ( 'NONE', #4609, #1453 ) ;
#6806=DIRECTION ( 'NONE',  ( -1.000000000000000000, 0.000000000000000000, 0.000000000000000000 ) ) ;
#6815=CIRCLE ( 'NONE', #19772, 11.99999999999998934 ) ;
#6849=CIRCLE ( 'NONE', #19815, 20.00000000000000000 ) ;
#6850=DIRECTION ( 'NONE',  ( 0.000000000000000000, -0.000000000000000000, 1.000000000000000000 ) ) ;
#6904=EDGE_LOOP ( 'NONE', ( #8334, #5852, #22899, #21413 ) ) ;
#6905=EDGE_CURVE ( 'NONE', #9950, #25953, #21083, .T. ) ;
#6907=FACE_OUTER_BOUND ( 'NONE', #19114, .T. ) ;
#6927=CIRCLE ( 'NONE', #8945, 15.00000000000000000 ) ;
#6942=ORIENTED_EDGE ( 'NONE', *, *, #6494, .F. ) ;
#6943=AXIS2_PLACEMENT_3D ( 'NONE', #13435, #8277, #5776 ) ;
#6952=EDGE_LOOP ( 'NONE', ( #1891, #15604, #15143, #13862 ) ) ;
#6981=CARTESIAN_POINT ( 'NONE',  ( 0.000000000000000000, 0.000000000000000000, -87.50000000000000000 ) ) ;
#6984=CARTESIAN_POINT ( 'NONE',  ( -50.00000000000000000, 0.000000000000000000, 196.3477631085023631 ) ) ;
#7032=CARTESIAN_POINT ( 'NONE',  ( 49.99999999999998579, -50.00000000000000000, -92.50000000000000000 ) ) ;
#7054=DIRECTION ( 'NONE',  ( 0.000000000000000000, 0.000000000000000000, -1.000000000000000000 ) ) ;
#7089=LINE ( 'NONE', #7714, #22333 ) ;
#7223=CARTESIAN_POINT ( 'NONE',  ( 0.000000000000000000, 0.000000000000000000, -87.50000000000000000 ) ) ;
#7225=ORIENTED_EDGE ( 'NONE', *, *, #1936, .T. ) ;
#7247=DIRECTION ( 'NONE',  ( 0.000000000000000000, 0.000000000000000000, 1.000000000000000000 ) ) ;
#7250=DIRECTION ( 'NONE',  ( -0.000000000000000000, -0.000000000000000000, -1.000000000000000000 ) ) ;
#7257=EDGE_CURVE ( 'NONE', #15581, #52, #15103, .T. ) ;
#7296=CARTESIAN_POINT ( 'NONE',  ( -12.73895949420588458, 48.35079126656098225, -47.06516019132716622 ) ) ;
#7321=DIRECTION ( 'NONE',  ( -1.000000000000000000, 0.000000000000000000, 0.000000000000000000 ) ) ;
#7327=CARTESIAN_POINT ( 'NONE',  ( 49.99999999999998579, 70.00000000000000000, 12.49999999999999112 ) ) ;
#7337=PLANE ( 'NONE',  #17111 ) ;
#7345=EDGE_LOOP ( 'NONE', ( #8673, #18697, #10268, #3041 ) ) ;
#7347=DIRECTION ( 'NONE',  ( 0.000000000000000000, 0.000000000000000000, -1.000000000000000000 ) ) ;
#7355=CARTESIAN_POINT ( 'NONE',  ( 0.000000000000000000, 0.000000000000000000, -52.50000000000000000 ) ) ;
#7392=CARTESIAN_POINT ( 'NONE',  ( 50.00000000000000000, 6.123233995736766085E-15, -87.50000000000000000 ) ) ;
#7396=AXIS2_PLACEMENT_3D ( 'NONE', #9486, #28514, #21014 ) ;
#7413=DIRECTION ( 'NONE',  ( 0.000000000000000000, 1.000000000000000000, 0.000000000000000000 ) ) ;
#7415=ORIENTED_EDGE ( 'NONE', *, *, #30363, .T. ) ;
#7427=ORIENTED_EDGE ( 'NONE', *, *, #7891, .T. ) ;
#7442=CARTESIAN_POINT ( 'NONE',  ( -50.00000000000000000, -70.00000000000000000, -92.50000000000000000 ) ) ;
#7460=AXIS2_PLACEMENT_3D ( 'NONE', #6272, #15784, #25306 ) ;
#7474=CIRCLE ( 'NONE', #26395, 20.00000000000000000 ) ;
#7476=ADVANCED_FACE ( 'NONE', ( #22444 ), #8581, .F. ) ;
#7488=DIRECTION ( 'NONE',  ( -1.000000000000000000, 0.000000000000000000, 0.000000000000000000 ) ) ;
#7501=VERTEX_POINT ( 'NONE', #12951 ) ;
#7510=EDGE_CURVE ( 'NONE', #20399, #4649, #22597, .T. ) ;
#7515=CARTESIAN_POINT ( 'NONE',  ( -70.00000000000000000, -70.00000000000000000, -92.50000000000000000 ) ) ;
#7516=CYLINDRICAL_SURFACE ( 'NONE', #25610, 11.99999999999998934 ) ;
#7537=DIRECTION ( 'NONE',  ( 0.000000000000000000, -1.000000000000000000, 0.000000000000000000 ) ) ;
#7551=CARTESIAN_POINT ( 'NONE',  ( -70.00000000000000000, -50.00000000000000000, -92.50000000000000000 ) ) ;
#7587=ORIENTED_EDGE ( 'NONE', *, *, #6905, .T. ) ;
#7654=ORIENTED_EDGE ( 'NONE', *, *, #30373, .T. ) ;
#7671=EDGE_CURVE ( 'NONE', #27143, #30053, #30239, .T. ) ;
#7679=ADVANCED_FACE ( 'NONE', ( #20034 ), #12719, .F. ) ;
#7681=CIRCLE ( 'NONE', #25110, 7.500000000000013323 ) ;
#7714=CARTESIAN_POINT ( 'NONE',  ( 50.00000000000000000, 6.123233995736766085E-15, 196.3477631085023631 ) ) ;
#7715=PLANE ( 'NONE',  #24045 ) ;
#7737=ORIENTED_EDGE ( 'NONE', *, *, #17620, .T. ) ;
#7753=PLANE ( 'NONE',  #2853 ) ;
#7762=FACE_OUTER_BOUND ( 'NONE', #22571, .T. ) ;
#7767=ORIENTED_EDGE ( 'NONE', *, *, #22560, .F. ) ;
#7779=DIRECTION ( 'NONE',  ( 0.000000000000000000, 0.000000000000000000, 1.000000000000000000 ) ) ;
#7795=DIRECTION ( 'NONE',  ( -1.000000000000000000, 0.000000000000000000, -0.000000000000000000 ) ) ;
#7798=EDGE_LOOP ( 'NONE', ( #24417, #15438, #28209, #12885, #25934, #21826, #11351, #2610, #29123, #8073 ) ) ;
#7810=AXIS2_PLACEMENT_3D ( 'NONE', #16304, #20105, #6635 ) ;
#7813=EDGE_CURVE ( 'NONE', #10221, #23441, #12565, .T. ) ;
#7815=EDGE_CURVE ( 'NONE', #28813, #9106, #22094, .T. ) ;
#7816=DIRECTION ( 'NONE',  ( 0.000000000000000000, 0.000000000000000000, -1.000000000000000000 ) ) ;
#7834=AXIS2_PLACEMENT_3D ( 'NONE', #26047, #9667, #26510 ) ;
#7843=CARTESIAN_POINT ( 'NONE',  ( 1.836970198721029589E-15, -14.99999999999997158, -70.00000000000000000 ) ) ;
#7848=AXIS2_PLACEMENT_3D ( 'NONE', #26689, #12813, #22311 ) ;
#7853=CARTESIAN_POINT ( 'NONE',  ( -50.00000000000000000, 0.000000000000000000, 12.49999999999998401 ) ) ;
#7865=CARTESIAN_POINT ( 'NONE',  ( -32.50000000000000000, 0.000000000000000000, -52.50000000000000000 ) ) ;
#7873=CARTESIAN_POINT ( 'NONE',  ( 0.000000000000000000, 0.000000000000000000, -87.50000000000000000 ) ) ;
#7886=DIRECTION ( 'NONE',  ( 0.000000000000000000, 0.000000000000000000, -1.000000000000000000 ) ) ;
#7891=EDGE_CURVE ( 'NONE', #30269, #27691, #11160, .T. ) ;
#7928=CARTESIAN_POINT ( 'NONE',  ( -5.311554845790392498, 49.71917005564084491, -40.96330688025074807 ) ) ;
#7960=ORIENTED_EDGE ( 'NONE', *, *, #15331, .T. ) ;
#8003=FACE_BOUND ( 'NONE', #26448, .T. ) ;
#8036=VERTEX_POINT ( 'NONE', #9104 ) ;
#8053=CARTESIAN_POINT ( 'NONE',  ( -37.99999999999999289, 70.00000000000000000, -34.49999999999999289 ) ) ;
#8073=ORIENTED_EDGE ( 'NONE', *, *, #5276, .T. ) ;
#8077=CARTESIAN_POINT ( 'NONE',  ( -7.943622683424091058, 49.36666681218739683, -67.73329464138640787 ) ) ;
#8094=EDGE_CURVE ( 'NONE', #6549, #17738, #14223, .T. ) ;
#8107=ORIENTED_EDGE ( 'NONE', *, *, #18151, .T. ) ;
#8133=DIRECTION ( 'NONE',  ( -1.000000000000000000, 0.000000000000000000, 0.000000000000000000 ) ) ;
#8134=CARTESIAN_POINT ( 'NONE',  ( -50.00000000000000000, -50.00000000000000000, 12.49999999999998401 ) ) ;
#8162=VERTEX_POINT ( 'NONE', #24364 ) ;
#8172=CARTESIAN_POINT ( 'NONE',  ( -37.99999999999999289, 209.2686044187655909, -40.50000000000000000 ) ) ;
#8195=CARTESIAN_POINT ( 'NONE',  ( -35.00000000000000000, 70.00000000000000000, -22.50000000000003908 ) ) ;
#8218=EDGE_CURVE ( 'NONE', #15437, #2838, #3009, .T. ) ;
#8224=CARTESIAN_POINT ( 'NONE',  ( -6.207687030005119233, 49.61523691829047067, -68.66397725790081097 ) ) ;
#8237=EDGE_LOOP ( 'NONE', ( #25594, #307 ) ) ;
#8265=DIRECTION ( 'NONE',  ( 0.000000000000000000, 0.000000000000000000, -1.000000000000000000 ) ) ;
#8266=CARTESIAN_POINT ( 'NONE',  ( 49.99999999999998579, 70.00000000000000000, -92.50000000000000000 ) ) ;
#8277=DIRECTION ( 'NONE',  ( 0.000000000000000000, 1.000000000000000000, -0.000000000000000000 ) ) ;
#8308=EDGE_CURVE ( 'NONE', #8162, #17860, #18871, .T. ) ;
#8322=LINE ( 'NONE', #14863, #21325 ) ;
#8325=CARTESIAN_POINT ( 'NONE',  ( -37.99999999999999289, 90.00000000000001421, -22.50000000000000711 ) ) ;
#8334=ORIENTED_EDGE ( 'NONE', *, *, #15462, .T. ) ;
#8390=AXIS2_PLACEMENT_3D ( 'NONE', #6248, #23069, #17961 ) ;
#8409=DIRECTION ( 'NONE',  ( 0.000000000000000000, 0.000000000000000000, -1.000000000000000000 ) ) ;
#8430=VERTEX_POINT ( 'NONE', #3413 ) ;
#8434=EDGE_CURVE ( 'NONE', #8903, #20793, #1074, .T. ) ;
#8441=CARTESIAN_POINT ( 'NONE',  ( -70.00000000000000000, 70.00000000000000000, -92.50000000000000000 ) ) ;
#8484=CARTESIAN_POINT ( 'NONE',  ( -37.99999999999999289, 90.00000000000001421, -34.49999999999999289 ) ) ;
#8558=VERTEX_POINT ( 'NONE', #27437 ) ;
#8559=CARTESIAN_POINT ( 'NONE',  ( 49.99999999999998579, -50.00000000000000000, -87.50000000000000000 ) ) ;
#8581=CYLINDRICAL_SURFACE ( 'NONE', #15128, 6.000000000000005329 ) ;
#8586=CARTESIAN_POINT ( 'NONE',  ( -57.50000000000001421, 50.00000000000000000, -87.50000000000000000 ) ) ;
#8610=CARTESIAN_POINT ( 'NONE',  ( 0.000000000000000000, 0.000000000000000000, -92.50000000000000000 ) ) ;
#8633=ADVANCED_FACE ( 'NONE', ( #2140 ), #1993, .F. ) ;
#8642=FACE_OUTER_BOUND ( 'NONE', #17003, .T. ) ;
#8673=ORIENTED_EDGE ( 'NONE', *, *, #12144, .T. ) ;
#8682=DIRECTION ( 'NONE',  ( 0.000000000000000000, 1.000000000000000000, 0.000000000000000000 ) ) ;
#8686=EDGE_LOOP ( 'NONE', ( #29054, #16429, #19970, #21482 ) ) ;
#8734=VERTEX_POINT ( 'NONE', #14458 ) ;
#8786=EDGE_CURVE ( 'NONE', #25279, #8903, #16291, .T. ) ;
#8802=CARTESIAN_POINT ( 'NONE',  ( -35.00000000000000000, 90.00000000000001421, -22.50000000000002487 ) ) ;
#8829=CARTESIAN_POINT ( 'NONE',  ( 38.00000000000000711, 209.2686044187655909, -22.50000000000002487 ) ) ;
#8853=VERTEX_POINT ( 'NONE', #9898 ) ;
#8896=PRODUCT_DEFINITION_CONTEXT ( 'detailed design', #4016, 'design' ) ;
#8903=VERTEX_POINT ( 'NONE', #14723 ) ;
#8917=FACE_BOUND ( 'NONE', #24843, .T. ) ;
#8938=CARTESIAN_POINT ( 'NONE',  ( -12.50000000000000000, 0.000000000000000000, -52.50000000000000000 ) ) ;
#8941=CARTESIAN_POINT ( 'NONE',  ( 13.46952963749417798, 48.15317560926965257, -61.67470994988012478 ) ) ;
#8945=AXIS2_PLACEMENT_3D ( 'NONE', #29433, #17571, #1044 ) ;
#8954=DIRECTION ( 'NONE',  ( -0.000000000000000000, -1.000000000000000000, -0.000000000000000000 ) ) ;
#8956=CIRCLE ( 'NONE', #6943, 6.000000000000005329 ) ;
#9015=EDGE_CURVE ( 'NONE', #2444, #15417, #9243, .T. ) ;
#9026=ADVANCED_FACE ( 'NONE', ( #6907 ), #23728, .F. ) ;
#9059=EDGE_LOOP ( 'NONE', ( #12103, #14009, #4559, #5815 ) ) ;
#9061=DIRECTION ( 'NONE',  ( -1.000000000000000000, 0.000000000000000000, -0.000000000000000000 ) ) ;
#9075=ORIENTED_EDGE ( 'NONE', *, *, #18908, .F. ) ;
#9094=CARTESIAN_POINT ( 'NONE',  ( 49.99999999999998579, 70.00000000000000000, -75.50000000000001421 ) ) ;
#9098=ORIENTED_EDGE ( 'NONE', *, *, #14936, .F. ) ;
#9104=CARTESIAN_POINT ( 'NONE',  ( -37.99999999999999289, 70.00000000000000000, -22.50000000000000711 ) ) ;
#9106=VERTEX_POINT ( 'NONE', #5179 ) ;
#9111=DIRECTION ( 'NONE',  ( 0.000000000000000000, 0.000000000000000000, -1.000000000000000000 ) ) ;
#9112=VERTEX_POINT ( 'NONE', #5958 ) ;
#9113=CARTESIAN_POINT ( 'NONE',  ( 1.868132521858655084E-15, 50.00000000000000000, -40.00000000000000711 ) ) ;
#9129=DIRECTION ( 'NONE',  ( 0.000000000000000000, 0.000000000000000000, 1.000000000000000000 ) ) ;
#9144=ORIENTED_EDGE ( 'NONE', *, *, #18908, .T. ) ;
#9148=ADVANCED_BREP_SHAPE_REPRESENTATION ( '', ( #3175, #7396 ), #9395 ) ;
#9155=CARTESIAN_POINT ( 'NONE',  ( 42.49999999999998579, 50.00000000000000000, -87.50000000000000000 ) ) ;
#9163=ADVANCED_FACE ( 'NONE', ( #8917, #20738 ), #4217, .F. ) ;
#9165=CIRCLE ( 'NONE', #26609, 7.500000000000000000 ) ;
#9167=DIRECTION ( 'NONE',  ( 0.000000000000000000, 0.000000000000000000, 1.000000000000000000 ) ) ;
#9180=ORIENTED_EDGE ( 'NONE', *, *, #19676, .T. ) ;
#9189=ADVANCED_FACE ( 'NONE', ( #16222 ), #23231, .F. ) ;
#9193=ADVANCED_FACE ( 'NONE', ( #10787 ), #30424, .T. ) ;
#9206=VECTOR ( 'NONE', #17193, 1000.000000000000000 ) ;
#9208=DIRECTION ( 'NONE',  ( 0.000000000000000000, -1.000000000000000000, 0.000000000000000000 ) ) ;
#9219=ADVANCED_FACE ( 'NONE', ( #4372 ), #13455, .T. ) ;
#9238=CARTESIAN_POINT ( 'NONE',  ( -37.99999999999999289, 209.2686044187655909, -87.50000000000000000 ) ) ;
#9243=LINE ( 'NONE', #25783, #6317 ) ;
#9247=EDGE_CURVE ( 'NONE', #23441, #23754, #3934, .T. ) ;
#9252=DIRECTION ( 'NONE',  ( -0.000000000000000000, -0.000000000000000000, 1.000000000000000000 ) ) ;
#9267=DIRECTION ( 'NONE',  ( 0.000000000000000000, 0.000000000000000000, 1.000000000000000000 ) ) ;
#9269=ORIENTED_EDGE ( 'NONE', *, *, #3767, .T. ) ;
#9286=DIRECTION ( 'NONE',  ( -0.000000000000000000, -0.000000000000000000, -1.000000000000000000 ) ) ;
#9293=CIRCLE ( 'NONE', #4810, 6.000000000000005329 ) ;
#9294=EDGE_LOOP ( 'NONE', ( #11241, #9324, #7427, #17158 ) ) ;
#9313=DIRECTION ( 'NONE',  ( -1.000000000000000000, 0.000000000000000000, 0.000000000000000000 ) ) ;
#9324=ORIENTED_EDGE ( 'NONE', *, *, #24003, .T. ) ;
#9333=EDGE_LOOP ( 'NONE', ( #19781, #6206 ) ) ;
#9349=ADVANCED_FACE ( 'NONE', ( #19338 ), #21188, .F. ) ;
#9360=VERTEX_POINT ( 'NONE', #26360 ) ;
#9370=CIRCLE ( 'NONE', #4379, 6.000000000000005329 ) ;
#9395=( GEOMETRIC_REPRESENTATION_CONTEXT ( 3 ) GLOBAL_UNCERTAINTY_ASSIGNED_CONTEXT ( ( #24168 ) ) GLOBAL_UNIT_ASSIGNED_CONTEXT ( ( #1361, #1054, #17726 ) ) REPRESENTATION_CONTEXT ( 'NONE', 'WORKASPACE' ) );
#9421=FACE_OUTER_BOUND ( 'NONE', #13709, .T. ) ;
#9436=DIRECTION ( 'NONE',  ( 0.000000000000000000, 0.000000000000000000, 1.000000000000000000 ) ) ;
#9444=DIRECTION ( 'NONE',  ( -0.000000000000000000, -0.000000000000000000, 1.000000000000000000 ) ) ;
#9452=LINE ( 'NONE', #26122, #15436 ) ;
#9476=DIRECTION ( 'NONE',  ( -0.000000000000000000, -0.000000000000000000, 1.000000000000000000 ) ) ;
#9480=ORIENTED_EDGE ( 'NONE', *, *, #21985, .T. ) ;
#9486=CARTESIAN_POINT ( 'NONE',  ( 0.000000000000000000, 0.000000000000000000, 0.000000000000000000 ) ) ;
#9533=CARTESIAN_POINT ( 'NONE',  ( 8.752233641273210907, 49.22975159878511420, -42.80828904653874645 ) ) ;
#9553=CARTESIAN_POINT ( 'NONE',  ( 42.49999999999998579, 50.00000000000000000, 52.07879600563550326 ) ) ;
#9588=PLANE ( 'NONE',  #29330 ) ;
#9605=ORIENTED_EDGE ( 'NONE', *, *, #21926, .T. ) ;
#9630=DIRECTION ( 'NONE',  ( 0.000000000000000000, 0.000000000000000000, 1.000000000000000000 ) ) ;
#9639=CARTESIAN_POINT ( 'NONE',  ( -13.44924491617056539, 48.15781802575228454, -61.66015067657107807 ) ) ;
#9642=EDGE_CURVE ( 'NONE', #25532, #9360, #20774, .T. ) ;
#9652=ORIENTED_EDGE ( 'NONE', *, *, #5062, .T. ) ;
#9667=DIRECTION ( 'NONE',  ( 0.000000000000000000, 0.000000000000000000, -1.000000000000000000 ) ) ;
#9732=DIRECTION ( 'NONE',  ( 0.000000000000000000, 0.000000000000000000, 1.000000000000000000 ) ) ;
#9742=ORIENTED_EDGE ( 'NONE', *, *, #19805, .T. ) ;
#9788=CARTESIAN_POINT ( 'NONE',  ( -8.751508360190436875, 49.22988072648480795, -42.80776806924027511 ) ) ;
#9815=CARTESIAN_POINT ( 'NONE',  ( 0.000000000000000000, 0.000000000000000000, -52.50000000000000000 ) ) ;
#9817=CARTESIAN_POINT ( 'NONE',  ( 0.000000000000000000, 90.00000000000001421, -55.00000000000000711 ) ) ;
#9825=DIRECTION ( 'NONE',  ( 0.000000000000000000, -0.000000000000000000, -1.000000000000000000 ) ) ;
#9838=EDGE_LOOP ( 'NONE', ( #23531, #30792, #18632, #9742, #9180, #9144, #6400, #30670, #10594, #7654 ) ) ;
#9848=FACE_OUTER_BOUND ( 'NONE', #12640, .T. ) ;
#9869=DIRECTION ( 'NONE',  ( -0.000000000000000000, -1.000000000000000000, -0.000000000000000000 ) ) ;
#9895=CARTESIAN_POINT ( 'NONE',  ( -37.99999999999999289, 209.2686044187655909, -87.50000000000000000 ) ) ;
#9898=CARTESIAN_POINT ( 'NONE',  ( 57.49999999999998579, -50.00000000000000000, 12.49999999999999112 ) ) ;
#9917=VECTOR ( 'NONE', #656, 1000.000000000000000 ) ;
#9923=EDGE_CURVE ( 'NONE', #1827, #23138, #23705, .T. ) ;
#9950=VERTEX_POINT ( 'NONE', #29068 ) ;
#9964=AXIS2_PLACEMENT_3D ( 'NONE', #19041, #12177, #26057 ) ;
#10007=CARTESIAN_POINT ( 'NONE',  ( 69.99999999999998579, 50.00000000000000000, -92.50000000000000000 ) ) ;
#10028=ORIENTED_EDGE ( 'NONE', *, *, #3704, .T. ) ;
#10037=ORIENTED_EDGE ( 'NONE', *, *, #21785, .T. ) ;
#10045=LINE ( 'NONE', #5365, #5396 ) ;
#10082=DIRECTION ( 'NONE',  ( 0.000000000000000000, 0.000000000000000000, -1.000000000000000000 ) ) ;
#10100=VECTOR ( 'NONE', #23279, 1000.000000000000000 ) ;
#10117=VERTEX_POINT ( 'NONE', #1755 ) ;
#10135=AXIS2_PLACEMENT_3D ( 'NONE', #29767, #8409, #17921 ) ;
#10151=DIRECTION ( 'NONE',  ( -1.000000000000000000, 0.000000000000000000, 0.000000000000000000 ) ) ;
#10182=VERTEX_POINT ( 'NONE', #19944 ) ;
#10193=FACE_OUTER_BOUND ( 'NONE', #26296, .T. ) ;
#10221=VERTEX_POINT ( 'NONE', #23351 ) ;
#10222=DIRECTION ( 'NONE',  ( 0.000000000000000000, 1.000000000000000000, 0.000000000000000000 ) ) ;
#10226=DIRECTION ( 'NONE',  ( -0.000000000000000000, -1.000000000000000000, -0.000000000000000000 ) ) ;
#10238=AXIS2_PLACEMENT_3D ( 'NONE', #25042, #19913, #10694 ) ;
#10250=VECTOR ( 'NONE', #7347, 1000.000000000000000 ) ;
#10268=ORIENTED_EDGE ( 'NONE', *, *, #25874, .T. ) ;
#10271=AXIS2_PLACEMENT_3D ( 'NONE', #26258, #5514, #14868 ) ;
#10272=FACE_OUTER_BOUND ( 'NONE', #6904, .T. ) ;
#10275=CARTESIAN_POINT ( 'NONE',  ( 0.000000000000000000, 90.00000000000001421, 0.000000000000000000 ) ) ;
#10283=AXIS2_PLACEMENT_3D ( 'NONE', #28036, #11655, #25697 ) ;
#10289=AXIS2_PLACEMENT_3D ( 'NONE', #16292, #30621, #9267 ) ;
#10292=VERTEX_POINT ( 'NONE', #30519 ) ;
#10295=ORIENTED_EDGE ( 'NONE', *, *, #14370, .T. ) ;
#10304=EDGE_LOOP ( 'NONE', ( #944, #273, #18809, #13084 ) ) ;
#10336=FACE_OUTER_BOUND ( 'NONE', #28192, .T. ) ;
#10353=ADVANCED_FACE ( 'NONE', ( #12439, #4635 ), #14136, .T. ) ;
#10388=DIRECTION ( 'NONE',  ( 0.000000000000000000, 0.000000000000000000, 1.000000000000000000 ) ) ;
#10390=LINE ( 'NONE', #29422, #17839 ) ;
#10392=CARTESIAN_POINT ( 'NONE',  ( 0.000000000000000000, 0.000000000000000000, -52.50000000000000000 ) ) ;
#10418=CARTESIAN_POINT ( 'NONE',  ( 12.50000000000000000, 1.530808498934191521E-15, -87.50000000000000000 ) ) ;
#10437=ORIENTED_EDGE ( 'NONE', *, *, #6494, .T. ) ;
#10439=CIRCLE ( 'NONE', #24891, 7.500000000000000000 ) ;
#10449=DIRECTION ( 'NONE',  ( -1.000000000000000000, 0.000000000000000000, 0.000000000000000000 ) ) ;
#10485=FACE_OUTER_BOUND ( 'NONE', #7798, .T. ) ;
#10487=PRODUCT_DEFINITION ( 'UNKNOWN', '', #23347, #8896 ) ;
#10543=ORIENTED_EDGE ( 'NONE', *, *, #24216, .F. ) ;
#10544=LINE ( 'NONE', #24895, #29249 ) ;
#10547=( LENGTH_UNIT ( ) NAMED_UNIT ( * ) SI_UNIT ( .MILLI., .METRE. ) );
#10578=CYLINDRICAL_SURFACE ( 'NONE', #24274, 6.000000000000005329 ) ;
#10594=ORIENTED_EDGE ( 'NONE', *, *, #11710, .T. ) ;
#10601=DIRECTION ( 'NONE',  ( -0.000000000000000000, -0.000000000000000000, 1.000000000000000000 ) ) ;
#10603=CARTESIAN_POINT ( 'NONE',  ( 57.49999999999998579, 50.00000000000000000, 52.07879600563550326 ) ) ;
#10624=CARTESIAN_POINT ( 'NONE',  ( 0.000000000000000000, 0.000000000000000000, -87.50000000000000000 ) ) ;
#10635=DIRECTION ( 'NONE',  ( 1.000000000000000000, 0.000000000000000000, 0.000000000000000000 ) ) ;
#10651=CARTESIAN_POINT ( 'NONE',  ( 14.97511466866788865, 47.70480676130072339, -55.99548085139268494 ) ) ;
#10657=DIRECTION ( 'NONE',  ( -0.000000000000000000, -1.000000000000000000, -0.000000000000000000 ) ) ;
#10694=DIRECTION ( 'NONE',  ( -1.000000000000000000, 0.000000000000000000, 0.000000000000000000 ) ) ;
#10710=CARTESIAN_POINT ( 'NONE',  ( -0.9831090015668330073, 49.99275926214126997, -69.97591847141403321 ) ) ;
#10779=ORIENTED_EDGE ( 'NONE', *, *, #25874, .F. ) ;
#10787=FACE_OUTER_BOUND ( 'NONE', #20565, .T. ) ;
#10812=CARTESIAN_POINT ( 'NONE',  ( 14.49323551690688383, 47.85361797699681574, -51.10247338586245291 ) ) ;
#10815=AXIS2_PLACEMENT_3D ( 'NONE', #14, #25757, #23246 ) ;
#10839=DIRECTION ( 'NONE',  ( 0.000000000000000000, 1.000000000000000000, -0.000000000000000000 ) ) ;
#10849=ORIENTED_EDGE ( 'NONE', *, *, #18588, .T. ) ;
#10864=LINE ( 'NONE', #5873, #6447 ) ;
#10894=CARTESIAN_POINT ( 'NONE',  ( 37.99999999999999289, 70.00000000000000000, -28.49999999999999645 ) ) ;
#10906=EDGE_CURVE ( 'NONE', #28482, #14635, #4330, .T. ) ;
#10951=DIRECTION ( 'NONE',  ( 0.000000000000000000, 0.000000000000000000, 1.000000000000000000 ) ) ;
#10975=CARTESIAN_POINT ( 'NONE',  ( 11.29805255599380587, 48.71189377371128160, -45.08539549253174528 ) ) ;
#10983=ORIENTED_EDGE ( 'NONE', *, *, #11235, .T. ) ;
#11013=AXIS2_PLACEMENT_3D ( 'NONE', #11269, #20764, #16550 ) ;
#11060=ADVANCED_FACE ( 'NONE', ( #20731 ), #27784, .F. ) ;
#11100=EDGE_CURVE ( 'NONE', #27407, #6185, #6273, .T. ) ;
#11130=EDGE_CURVE ( 'NONE', #23754, #13645, #19185, .T. ) ;
#11160=CIRCLE ( 'NONE', #12151, 11.99999999999998224 ) ;
#11203=ORIENTED_EDGE ( 'NONE', *, *, #29175, .T. ) ;
#11205=LINE ( 'NONE', #13413, #15748 ) ;
#11207=VERTEX_POINT ( 'NONE', #8586 ) ;
#11235=EDGE_CURVE ( 'NONE', #52, #946, #12797, .T. ) ;
#11241=ORIENTED_EDGE ( 'NONE', *, *, #8786, .F. ) ;
#11269=CARTESIAN_POINT ( 'NONE',  ( -50.00000000000000000, 50.00000000000000000, -87.50000000000000000 ) ) ;
#11272=AXIS2_PLACEMENT_3D ( 'NONE', #2606, #26786, #5412 ) ;
#11351=ORIENTED_EDGE ( 'NONE', *, *, #8094, .F. ) ;
#11379=CARTESIAN_POINT ( 'NONE',  ( -37.99999999999999289, 209.2686044187655909, -28.49999999999998934 ) ) ;
#11388=AXIS2_PLACEMENT_3D ( 'NONE', #1086, #10601, #3897 ) ;
#11396=AXIS2_PLACEMENT_3D ( 'NONE', #17160, #11461, #9111 ) ;
#11450=DIRECTION ( 'NONE',  ( -1.000000000000000000, 0.000000000000000000, 0.000000000000000000 ) ) ;
#11461=DIRECTION ( 'NONE',  ( -0.000000000000000000, -1.000000000000000000, -0.000000000000000000 ) ) ;
#11463=DIRECTION ( 'NONE',  ( 0.000000000000000000, 0.000000000000000000, -1.000000000000000000 ) ) ;
#11495=EDGE_CURVE ( 'NONE', #8162, #28813, #16818, .T. ) ;
#11518=CARTESIAN_POINT ( 'NONE',  ( 0.000000000000000000, 0.000000000000000000, -87.50000000000000000 ) ) ;
#11528=DIRECTION ( 'NONE',  ( 0.000000000000000000, 0.000000000000000000, -1.000000000000000000 ) ) ;
#11539=AXIS2_PLACEMENT_3D ( 'NONE', #30667, #4490, #2607 ) ;
#11598=CARTESIAN_POINT ( 'NONE',  ( 49.99999999999998579, 50.00000000000000000, 52.07879600563550326 ) ) ;
#11607=DIRECTION ( 'NONE',  ( 0.000000000000000000, 0.000000000000000000, 1.000000000000000000 ) ) ;
#11655=DIRECTION ( 'NONE',  ( 0.000000000000000000, 1.000000000000000000, 0.000000000000000000 ) ) ;
#11662=CARTESIAN_POINT ( 'NONE',  ( -37.99999999999999289, 209.2686044187655909, -75.50000000000000000 ) ) ;
#11667=EDGE_CURVE ( 'NONE', #11816, #11851, #25219, .T. ) ;
#11677=AXIS2_PLACEMENT_3D ( 'NONE', #17774, #22291, #3583 ) ;
#11709=VERTEX_POINT ( 'NONE', #5351 ) ;
#11710=EDGE_CURVE ( 'NONE', #10221, #6658, #12379, .T. ) ;
#11732=AXIS2_PLACEMENT_3D ( 'NONE', #3939, #18274, #27797 ) ;
#11782=EDGE_LOOP ( 'NONE', ( #21921, #23222, #676, #4352 ) ) ;
#11804=DIRECTION ( 'NONE',  ( 1.000000000000000000, 0.000000000000000000, -0.000000000000000000 ) ) ;
#11816=VERTEX_POINT ( 'NONE', #19543 ) ;
#11830=B_SPLINE_CURVE_WITH_KNOTS ( 'NONE', 3,
 ( #24440, #24288, #2616, #19755, #26800, #29285, #7928, #5427, #19455, #9788, #19305, #16809, #26954, #21793, #28973, #7296, #14297, #23816, #17113, #19606, #12136, #26323, #26637, #2937, #4957, #12455, #21945, #572, #272, #14930, #3080, #2466, #9639, #11984, #26477, #118, #19151, #14623, #28666, #2775, #1053, #8077, #22411, #3388, #8224, #5576, #20071, #29908, #29591, #10710, #15215, #22252 ),
 .UNSPECIFIED., .F., .F.,
 ( 4, 2, 2, 2, 2, 2, 2, 2, 2, 2, 2, 2, 2, 2, 2, 2, 2, 2, 2, 2, 2, 2, 2, 2, 2, 4 ),
 ( 1.813955208755348987E-18, 0.002948126770087892892, 0.004422190155131839120, 0.005896253540175785783, 0.008844380310263671302, 0.01031844369530762057, 0.01179250708035156983, 0.01474063385043945969, 0.01621469723548340028, 0.01768876062052733913, 0.01916282400557127452, 0.02063688739061521338, 0.02358501416070309109, 0.02505907754574704382, 0.02653314093079099656, 0.02948126770087891590, 0.03095533108592286517, 0.03242939447096682831, 0.03390345785601079492, 0.03537752124105476154, 0.03832564801114272945, 0.03979971139618670994, 0.04127377478123069043, 0.04422190155131865141, 0.04569596493636263884, 0.04717002832140662627 ),
 .UNSPECIFIED. ) ;
#11841=EDGE_CURVE ( 'NONE', #8036, #13645, #14702, .T. ) ;
#11851=VERTEX_POINT ( 'NONE', #7392 ) ;
#11854=CARTESIAN_POINT ( 'NONE',  ( 0.000000000000000000, 0.000000000000000000, 196.3477631085023631 ) ) ;
#11877=DIRECTION ( 'NONE',  ( -1.000000000000000000, 0.000000000000000000, 0.000000000000000000 ) ) ;
#11926=AXIS2_PLACEMENT_3D ( 'NONE', #14429, #7413, #12095 ) ;
#11940=ADVANCED_FACE ( 'NONE', ( #18137 ), #5817, .F. ) ;
#11943=DIRECTION ( 'NONE',  ( 0.000000000000000000, 0.000000000000000000, 1.000000000000000000 ) ) ;
#11954=CARTESIAN_POINT ( 'NONE',  ( -42.49999999999998579, -50.00000000000000000, 52.07879600563550326 ) ) ;
#11978=CYLINDRICAL_SURFACE ( 'NONE', #6290, 11.99999999999999645 ) ;
#11984=CARTESIAN_POINT ( 'NONE',  ( -12.98621692273268913, 48.28473667581032913, -62.52316196060546361 ) ) ;
#12036=CARTESIAN_POINT ( 'NONE',  ( 3.903322525700887002, 49.84968173887558152, -40.50827906751979413 ) ) ;
#12057=VERTEX_POINT ( 'NONE', #28560 ) ;
#12067=ORIENTED_EDGE ( 'NONE', *, *, #18492, .F. ) ;
#12095=DIRECTION ( 'NONE',  ( 0.000000000000000000, 0.000000000000000000, 1.000000000000000000 ) ) ;
#12103=ORIENTED_EDGE ( 'NONE', *, *, #26915, .F. ) ;
#12107=ADVANCED_FACE ( 'NONE', ( #12343 ), #2664, .T. ) ;
#12136=CARTESIAN_POINT ( 'NONE',  ( -14.20303051544474826, 47.94055110225200167, -50.15062527444063534 ) ) ;
#12137=AXIS2_PLACEMENT_3D ( 'NONE', #18444, #20903, #4078 ) ;
#12144=EDGE_CURVE ( 'NONE', #10182, #8853, #10439, .T. ) ;
#12151=AXIS2_PLACEMENT_3D ( 'NONE', #27837, #10839, #1777 ) ;
#12161=DIRECTION ( 'NONE',  ( -0.000000000000000000, -0.000000000000000000, -1.000000000000000000 ) ) ;
#12177=DIRECTION ( 'NONE',  ( 0.000000000000000000, 1.000000000000000000, 0.000000000000000000 ) ) ;
#12210=CARTESIAN_POINT ( 'NONE',  ( -35.00000000000000000, 70.00000000000000000, 12.49999999999999112 ) ) ;
#12219=EDGE_CURVE ( 'NONE', #16188, #13747, #8956, .T. ) ;
#12226=CARTESIAN_POINT ( 'NONE',  ( -37.99999999999999289, 70.00000000000000000, -75.50000000000000000 ) ) ;
#12326=AXIS2_PLACEMENT_3D ( 'NONE', #8134, #17016, #10151 ) ;
#12343=FACE_OUTER_BOUND ( 'NONE', #10304, .T. ) ;
#12352=AXIS2_PLACEMENT_3D ( 'NONE', #905, #5733, #3092 ) ;
#12373=CIRCLE ( 'NONE', #18853, 50.00000000000000000 ) ;
#12375=CARTESIAN_POINT ( 'NONE',  ( -70.00000000000000000, -70.00000000000000000, -92.50000000000000000 ) ) ;
#12376=DIRECTION ( 'NONE',  ( -0.000000000000000000, -1.000000000000000000, -0.000000000000000000 ) ) ;
#12377=ORIENTED_EDGE ( 'NONE', *, *, #23477, .T. ) ;
#12379=LINE ( 'NONE', #26886, #22231 ) ;
#12391=ORIENTED_EDGE ( 'NONE', *, *, #3877, .T. ) ;
#12414=ORIENTED_EDGE ( 'NONE', *, *, #7510, .F. ) ;
#12419=EDGE_CURVE ( 'NONE', #26519, #23441, #18045, .T. ) ;
#12439=FACE_OUTER_BOUND ( 'NONE', #9333, .T. ) ;
#12441=CYLINDRICAL_SURFACE ( 'NONE', #11272, 6.000000000000005329 ) ;
#12444=FACE_OUTER_BOUND ( 'NONE', #8686, .T. ) ;
#12455=CARTESIAN_POINT ( 'NONE',  ( -15.00022444080144091, 47.69688948748883206, -55.48551676194295368 ) ) ;
#12507=CIRCLE ( 'NONE', #11013, 7.500000000000013323 ) ;
#12522=DIRECTION ( 'NONE',  ( -1.000000000000000000, 0.000000000000000000, 0.000000000000000000 ) ) ;
#12565=LINE ( 'NONE', #693, #21606 ) ;
#12600=DIRECTION ( 'NONE',  ( 0.000000000000000000, -0.000000000000000000, -1.000000000000000000 ) ) ;
#12607=ORIENTED_EDGE ( 'NONE', *, *, #3704, .F. ) ;
#12613=ORIENTED_EDGE ( 'NONE', *, *, #12681, .T. ) ;
#12618=EDGE_CURVE ( 'NONE', #25532, #21023, #9452, .T. ) ;
#12635=ORIENTED_EDGE ( 'NONE', *, *, #7510, .T. ) ;
#12640=EDGE_LOOP ( 'NONE', ( #15903, #16998, #15381, #26816 ) ) ;
#12681=EDGE_CURVE ( 'NONE', #17738, #946, #23937, .T. ) ;
#12700=FACE_OUTER_BOUND ( 'NONE', #9294, .T. ) ;
#12704=FACE_OUTER_BOUND ( 'NONE', #17436, .T. ) ;
#12712=DIRECTION ( 'NONE',  ( -0.000000000000000000, 0.000000000000000000, 1.000000000000000000 ) ) ;
#12719=PLANE ( 'NONE',  #13660 ) ;
#12723=LINE ( 'NONE', #24710, #5228 ) ;
#12741=CARTESIAN_POINT ( 'NONE',  ( 35.00000000000000000, 90.00000000000001421, -22.50000000000002487 ) ) ;
#12763=FACE_OUTER_BOUND ( 'NONE', #22711, .T. ) ;
#12797=LINE ( 'NONE', #5625, #25190 ) ;
#12809=AXIS2_PLACEMENT_3D ( 'NONE', #1728, #1885, #20900 ) ;
#12813=DIRECTION ( 'NONE',  ( -0.000000000000000000, -1.000000000000000000, -0.000000000000000000 ) ) ;
#12861=DIRECTION ( 'NONE',  ( 0.000000000000000000, 1.000000000000000000, 0.000000000000000000 ) ) ;
#12866=AXIS2_PLACEMENT_3D ( 'NONE', #13735, #20450, #10951 ) ;
#12885=ORIENTED_EDGE ( 'NONE', *, *, #20, .T. ) ;
#12903=LINE ( 'NONE', #29430, #20715 ) ;
#12921=EDGE_LOOP ( 'NONE', ( #13822, #6942 ) ) ;
#12951=CARTESIAN_POINT ( 'NONE',  ( -37.99999999999999289, 90.00000000000001421, -40.50000000000000000 ) ) ;
#12986=DIRECTION ( 'NONE',  ( -1.000000000000000000, 0.000000000000000000, -0.000000000000000000 ) ) ;
#13003=CARTESIAN_POINT ( 'NONE',  ( 1.837104849652355830E-15, 50.00000000000000000, -70.00000000000000000 ) ) ;
#13068=ORIENTED_EDGE ( 'NONE', *, *, #5389, .F. ) ;
#13082=VECTOR ( 'NONE', #1627, 1000.000000000000000 ) ;
#13084=ORIENTED_EDGE ( 'NONE', *, *, #29150, .T. ) ;
#13113=VERTEX_POINT ( 'NONE', #30158 ) ;
#13125=LINE ( 'NONE', #5947, #18313 ) ;
#13154=CARTESIAN_POINT ( 'NONE',  ( 0.4912064067415030100, 50.00000000000000000, -70.00000000000001421 ) ) ;
#13196=FACE_OUTER_BOUND ( 'NONE', #19163, .T. ) ;
#13213=DIRECTION ( 'NONE',  ( 1.000000000000000000, 0.000000000000000000, -1.369518533665900065E-16 ) ) ;
#13274=AXIS2_PLACEMENT_3D ( 'NONE', #26632, #26948, #3073 ) ;
#13319=CARTESIAN_POINT ( 'NONE',  ( 49.99999999999998579, -50.00000000000000000, -87.50000000000000000 ) ) ;
#13351=VECTOR ( 'NONE', #25778, 1000.000000000000000 ) ;
#13355=DIRECTION ( 'NONE',  ( -0.000000000000000000, 1.000000000000000000, -0.000000000000000000 ) ) ;
#13407=ADVANCED_FACE ( 'NONE', ( #10485, #27176, #20460, #29365, #29980, #8003 ), #26875, .F. ) ;
#13413=CARTESIAN_POINT ( 'NONE',  ( -70.00000000000000000, 50.00000000000000000, -92.50000000000000000 ) ) ;
#13435=CARTESIAN_POINT ( 'NONE',  ( -37.99999999999999289, 70.00000000000000000, -34.49999999999999289 ) ) ;
#13447=EDGE_LOOP ( 'NONE', ( #23212, #18698 ) ) ;
#13450=CARTESIAN_POINT ( 'NONE',  ( -49.99999999999998579, 209.2686044187655909, -75.50000000000002842 ) ) ;
#13453=ORIENTED_EDGE ( 'NONE', *, *, #30177, .T. ) ;
#13455=CYLINDRICAL_SURFACE ( 'NONE', #27770, 20.00000000000000355 ) ;
#13459=DIRECTION ( 'NONE',  ( 0.000000000000000000, 0.000000000000000000, -1.000000000000000000 ) ) ;
#13505=LINE ( 'NONE', #8195, #15828 ) ;
#13507=ORIENTED_EDGE ( 'NONE', *, *, #1592, .F. ) ;
#13508=CARTESIAN_POINT ( 'NONE',  ( 42.49999999999998579, -50.00000000000000000, 52.07879600563550326 ) ) ;
#13592=DIRECTION ( 'NONE',  ( 0.000000000000000000, 0.000000000000000000, -1.000000000000000000 ) ) ;
#13628=CARTESIAN_POINT ( 'NONE',  ( 9.913295469302216389, 49.01253027209195778, -66.29974890224383444 ) ) ;
#13637=CARTESIAN_POINT ( 'NONE',  ( -70.00000000000000000, -70.00000000000000000, 12.49999999999999112 ) ) ;
#13645=VERTEX_POINT ( 'NONE', #3547 ) ;
#13647=DIRECTION ( 'NONE',  ( -1.369518533665900065E-16, 0.000000000000000000, -1.000000000000000000 ) ) ;
#13660=AXIS2_PLACEMENT_3D ( 'NONE', #22216, #5231, #5688 ) ;
#13694=PLANE ( 'NONE',  #28266 ) ;
#13709=EDGE_LOOP ( 'NONE', ( #12414, #16726, #7587, #3055 ) ) ;
#13720=ORIENTED_EDGE ( 'NONE', *, *, #2378, .T. ) ;
#13735=CARTESIAN_POINT ( 'NONE',  ( 37.99999999999999289, 70.00000000000000000, -34.50000000000000000 ) ) ;
#13738=ORIENTED_EDGE ( 'NONE', *, *, #1590, .F. ) ;
#13739=DIRECTION ( 'NONE',  ( 0.000000000000000000, 0.000000000000000000, -1.000000000000000000 ) ) ;
#13740=DIRECTION ( 'NONE',  ( -1.000000000000000000, 0.000000000000000000, 0.000000000000000000 ) ) ;
#13746=DIRECTION ( 'NONE',  ( 1.000000000000000000, 0.000000000000000000, 0.000000000000000000 ) ) ;
#13747=VERTEX_POINT ( 'NONE', #30360 ) ;
#13754=ORIENTED_EDGE ( 'NONE', *, *, #17730, .T. ) ;
#13759=APPLICATION_CONTEXT ( 'automotive_design' ) ;
#13761=CARTESIAN_POINT ( 'NONE',  ( 1.977841715212117935, 49.97021211411167485, -40.09845259988525612 ) ) ;
#13821=ORIENTED_EDGE ( 'NONE', *, *, #30763, .F. ) ;
#13822=ORIENTED_EDGE ( 'NONE', *, *, #23824, .F. ) ;
#13826=DIRECTION ( 'NONE',  ( -0.000000000000000000, -1.000000000000000000, -0.000000000000000000 ) ) ;
#13833=ORIENTED_EDGE ( 'NONE', *, *, #16472, .F. ) ;
#13862=ORIENTED_EDGE ( 'NONE', *, *, #17730, .F. ) ;
#13879=LINE ( 'NONE', #30555, #2126 ) ;
#13912=ORIENTED_EDGE ( 'NONE', *, *, #23824, .T. ) ;
#13944=ADVANCED_FACE ( 'NONE', ( #27213 ), #17866, .F. ) ;
#14009=ORIENTED_EDGE ( 'NONE', *, *, #9015, .T. ) ;
#14019=VECTOR ( 'NONE', #5129, 1000.000000000000000 ) ;
#14034=ORIENTED_EDGE ( 'NONE', *, *, #8218, .T. ) ;
#14037=FACE_OUTER_BOUND ( 'NONE', #5546, .T. ) ;
#14047=ORIENTED_EDGE ( 'NONE', *, *, #17830, .T. ) ;
#14089=CARTESIAN_POINT ( 'NONE',  ( -37.99999999999999289, 90.00000000000001421, -34.49999999999999289 ) ) ;
#14136=PLANE ( 'NONE',  #23215 ) ;
#14137=ADVANCED_FACE ( 'NONE', ( #660 ), #19219, .F. ) ;
#14161=AXIS2_PLACEMENT_3D ( 'NONE', #6538, #20711, #15906 ) ;
#14200=ORIENTED_EDGE ( 'NONE', *, *, #12681, .F. ) ;
#14207=ORIENTED_EDGE ( 'NONE', *, *, #20809, .T. ) ;
#14223=LINE ( 'NONE', #23736, #30507 ) ;
#14263=CIRCLE ( 'NONE', #10289, 11.99999999999999645 ) ;
#14285=DIRECTION ( 'NONE',  ( -0.000000000000000000, -0.000000000000000000, -1.000000000000000000 ) ) ;
#14296=AXIS2_PLACEMENT_3D ( 'NONE', #24228, #24077, #11943 ) ;
#14297=CARTESIAN_POINT ( 'NONE',  ( -12.99194183819582449, 48.28319231324876171, -47.48680334385887392 ) ) ;
#14322=VECTOR ( 'NONE', #16225, 1000.000000000000000 ) ;
#14364=CARTESIAN_POINT ( 'NONE',  ( 49.99999999999998579, -50.00000000000000000, 12.49999999999999112 ) ) ;
#14370=EDGE_CURVE ( 'NONE', #4649, #25953, #25085, .T. ) ;
#14401=CYLINDRICAL_SURFACE ( 'NONE', #1249, 7.500000000000000000 ) ;
#14418=DIRECTION ( 'NONE',  ( 0.000000000000000000, 1.000000000000000000, 0.000000000000000000 ) ) ;
#14429=CARTESIAN_POINT ( 'NONE',  ( 37.99999999999999289, 90.00000000000001421, -34.50000000000000000 ) ) ;
#14445=VECTOR ( 'NONE', #13213, 1000.000000000000000 ) ;
#14458=CARTESIAN_POINT ( 'NONE',  ( -37.99999999999999289, 90.00000000000001421, -81.50000000000000000 ) ) ;
#14499=ORIENTED_EDGE ( 'NONE', *, *, #5602, .F. ) ;
#14515=ADVANCED_FACE ( 'NONE', ( #14037 ), #7337, .F. ) ;
#14533=EDGE_CURVE ( 'NONE', #17860, #17738, #3678, .T. ) ;
#14559=ORIENTED_EDGE ( 'NONE', *, *, #23783, .T. ) ;
#14584=EDGE_LOOP ( 'NONE', ( #7225, #26900, #2267, #689, #5584 ) ) ;
#14600=VECTOR ( 'NONE', #10657, 1000.000000000000000 ) ;
#14623=CARTESIAN_POINT ( 'NONE',  ( -11.28151912705817672, 48.71169459815545366, -64.89780961319154073 ) ) ;
#14635=VERTEX_POINT ( 'NONE', #14652 ) ;
#14652=CARTESIAN_POINT ( 'NONE',  ( 37.99999999999999289, 90.00000000000001421, -81.50000000000001421 ) ) ;
#14702=LINE ( 'NONE', #2859, #319 ) ;
#14723=CARTESIAN_POINT ( 'NONE',  ( 38.00000000000000711, 90.00000000000001421, -87.50000000000000000 ) ) ;
#14729=CARTESIAN_POINT ( 'NONE',  ( 35.00000000000000000, 70.00000000000000000, -22.50000000000003908 ) ) ;
#14794=FACE_OUTER_BOUND ( 'NONE', #3770, .T. ) ;
#14798=CARTESIAN_POINT ( 'NONE',  ( -50.00000000000000000, -50.00000000000000000, 52.07879600563550326 ) ) ;
#14800=FACE_BOUND ( 'NONE', #19955, .T. ) ;
#14816=CARTESIAN_POINT ( 'NONE',  ( 57.49999999999998579, -50.00000000000000000, -87.50000000000000000 ) ) ;
#14825=VECTOR ( 'NONE', #27552, 1000.000000000000000 ) ;
#14863=CARTESIAN_POINT ( 'NONE',  ( -32.50000000000000000, 0.000000000000000000, -52.50000000000000000 ) ) ;
#14867=DIRECTION ( 'NONE',  ( -0.000000000000000000, -1.000000000000000000, -0.000000000000000000 ) ) ;
#14868=DIRECTION ( 'NONE',  ( -1.000000000000000000, 0.000000000000000000, 0.000000000000000000 ) ) ;
#14922=EDGE_CURVE ( 'NONE', #52, #6549, #16500, .T. ) ;
#14930=CARTESIAN_POINT ( 'NONE',  ( -14.51554025688286309, 47.84704637152103857, -58.90721167866684738 ) ) ;
#14936=EDGE_CURVE ( 'NONE', #13113, #10117, #4156, .T. ) ;
#14981=CARTESIAN_POINT ( 'NONE',  ( -50.00000000000000000, -50.00000000000000000, -87.50000000000000000 ) ) ;
#15010=ORIENTED_EDGE ( 'NONE', *, *, #22919, .F. ) ;
#15033=CARTESIAN_POINT ( 'NONE',  ( 69.99999999999998579, -50.00000000000000000, -92.50000000000000000 ) ) ;
#15078=CARTESIAN_POINT ( 'NONE',  ( 57.49999999999998579, 50.00000000000000000, 12.49999999999999112 ) ) ;
#15081=ORIENTED_EDGE ( 'NONE', *, *, #24216, .T. ) ;
#15095=CARTESIAN_POINT ( 'NONE',  ( -50.00000000000000000, 70.00000000000000000, -92.50000000000000000 ) ) ;
#15103=CIRCLE ( 'NONE', #12137, 20.00000000000000000 ) ;
#15105=DIRECTION ( 'NONE',  ( 0.000000000000000000, 0.000000000000000000, 1.000000000000000000 ) ) ;
#15128=AXIS2_PLACEMENT_3D ( 'NONE', #24788, #6226, #1554 ) ;
#15143=ORIENTED_EDGE ( 'NONE', *, *, #1592, .T. ) ;
#15152=ORIENTED_EDGE ( 'NONE', *, *, #19528, .F. ) ;
#15153=ADVANCED_FACE ( 'NONE', ( #20216 ), #15541, .T. ) ;
#15166=CYLINDRICAL_SURFACE ( 'NONE', #827, 11.99999999999998224 ) ;
#15215=CARTESIAN_POINT ( 'NONE',  ( -0.4913386815044658573, 49.99999999999999289, -70.00000000000001421 ) ) ;
#15301=FACE_OUTER_BOUND ( 'NONE', #20967, .T. ) ;
#15322=CARTESIAN_POINT ( 'NONE',  ( 14.80383744458522877, 47.75831397104769849, -57.46711200187744595 ) ) ;
#15331=EDGE_CURVE ( 'NONE', #9950, #20399, #18147, .T. ) ;
#15343=ORIENTED_EDGE ( 'NONE', *, *, #28350, .T. ) ;
#15363=DIRECTION ( 'NONE',  ( 0.000000000000000000, 0.000000000000000000, 1.000000000000000000 ) ) ;
#15380=AXIS2_PLACEMENT_3D ( 'NONE', #5498, #24512, #12986 ) ;
#15381=ORIENTED_EDGE ( 'NONE', *, *, #28461, .T. ) ;
#15412=B_SPLINE_CURVE_WITH_KNOTS ( 'NONE', 3,
 ( #13003, #13154, #23106, #29681, #5979, #24851, #22492, #15789, #27816, #6443, #22646, #25474, #13628, #3957, #3792, #1751, #30294, #1139, #8941, #5822, #15479, #15322, #1297, #10651, #25312, #22813, #20162, #17996, #10812, #27504, #20326, #29851, #1464, #6124, #10975, #20475, #25624, #19049, #9533, #28415, #26067, #4239, #16548, #12036, #30443, #13761, #2361, #4698 ),
 .UNSPECIFIED., .F., .F.,
 ( 4, 2, 2, 2, 2, 2, 2, 2, 2, 2, 2, 2, 2, 2, 2, 2, 2, 2, 2, 2, 2, 2, 2, 4 ),
 ( 0.04717002832140662627, 0.04864369486941700488, 0.05011736141742738349, 0.05306469451344814070, 0.05453836106145851931, 0.05601202760946889792, 0.05895936070548962737, 0.06043302725349997823, 0.06190669380151032214, 0.06485402689753103078, 0.06780135999355173249, 0.06927502654156207640, 0.07074869308957243419, 0.07369602618559310814, 0.07516969273360343817, 0.07664335928161378209, 0.07959069237763446991, 0.08253802547365514386, 0.08401169202166547390, 0.08548535856967581781, 0.08843269166569647788, 0.08990635821370680791, 0.09138002476171713795, 0.09432735785773779802 ),
 .UNSPECIFIED. ) ;
#15417=VERTEX_POINT ( 'NONE', #30313 ) ;
#15423=FACE_OUTER_BOUND ( 'NONE', #16072, .T. ) ;
#15436=VECTOR ( 'NONE', #9286, 1000.000000000000000 ) ;
#15437=VERTEX_POINT ( 'NONE', #28131 ) ;
#15438=ORIENTED_EDGE ( 'NONE', *, *, #9923, .T. ) ;
#15439=ADVANCED_FACE ( 'NONE', ( #25642 ), #6464, .F. ) ;
#15458=EDGE_CURVE ( 'NONE', #20399, #9950, #9165, .T. ) ;
#15462=EDGE_CURVE ( 'NONE', #8558, #27143, #7681, .T. ) ;
#15471=VERTEX_POINT ( 'NONE', #3428 ) ;
#15479=CARTESIAN_POINT ( 'NONE',  ( 14.51487557364575842, 47.84724665906151131, -58.90888295343145131 ) ) ;
#15482=ADVANCED_FACE ( 'NONE', ( #1248 ), #29160, .F. ) ;
#15491=ADVANCED_FACE ( 'NONE', ( #15423 ), #22445, .F. ) ;
#15506=EDGE_LOOP ( 'NONE', ( #13833, #1787, #30685, #19461 ) ) ;
#15541=CYLINDRICAL_SURFACE ( 'NONE', #698, 20.00000000000000000 ) ;
#15547=EDGE_CURVE ( 'NONE', #25953, #4649, #29116, .T. ) ;
#15550=DIRECTION ( 'NONE',  ( -0.000000000000000000, -1.000000000000000000, -0.000000000000000000 ) ) ;
#15581=VERTEX_POINT ( 'NONE', #8266 ) ;
#15604=ORIENTED_EDGE ( 'NONE', *, *, #20656, .F. ) ;
#15609=EDGE_LOOP ( 'NONE', ( #17622, #18468, #2357, #9269, #5969, #18195 ) ) ;
#15654=EDGE_CURVE ( 'NONE', #2838, #25122, #20143, .T. ) ;
#15667=EDGE_CURVE ( 'NONE', #12057, #13747, #30089, .T. ) ;
#15688=CARTESIAN_POINT ( 'NONE',  ( -37.99999999999999289, 90.00000000000001421, -22.50000000000001421 ) ) ;
#15689=DIRECTION ( 'NONE',  ( 1.000000000000000000, 0.000000000000000000, 0.000000000000000000 ) ) ;
#15748=VECTOR ( 'NONE', #1544, 1000.000000000000000 ) ;
#15757=DIRECTION ( 'NONE',  ( -1.000000000000000000, 0.000000000000000000, -0.000000000000000000 ) ) ;
#15784=DIRECTION ( 'NONE',  ( -0.000000000000000000, 1.000000000000000000, -0.000000000000000000 ) ) ;
#15789=CARTESIAN_POINT ( 'NONE',  ( 6.209160252570208982, 49.61505262654815596, -68.66330880567365114 ) ) ;
#15828=VECTOR ( 'NONE', #30171, 1000.000000000000000 ) ;
#15870=EDGE_LOOP ( 'NONE', ( #19645, #13754 ) ) ;
#15874=CARTESIAN_POINT ( 'NONE',  ( -50.00000000000000000, 50.00000000000000000, 12.49999999999999112 ) ) ;
#15885=VECTOR ( 'NONE', #20860, 1000.000000000000000 ) ;
#15903=ORIENTED_EDGE ( 'NONE', *, *, #30373, .F. ) ;
#15906=DIRECTION ( 'NONE',  ( 0.000000000000000000, 0.000000000000000000, 1.000000000000000000 ) ) ;
#15911=CARTESIAN_POINT ( 'NONE',  ( -50.00000000000000000, 70.00000000000000000, -34.49999999999999289 ) ) ;
#15945=VECTOR ( 'NONE', #7250, 1000.000000000000000 ) ;
#16072=EDGE_LOOP ( 'NONE', ( #661, #6156 ) ) ;
#16138=CIRCLE ( 'NONE', #2688, 7.500000000000013323 ) ;
#16188=VERTEX_POINT ( 'NONE', #24556 ) ;
#16192=DIRECTION ( 'NONE',  ( 0.000000000000000000, 1.000000000000000000, -0.000000000000000000 ) ) ;
#16213=EDGE_CURVE ( 'NONE', #24252, #1827, #12723, .T. ) ;
#16222=FACE_OUTER_BOUND ( 'NONE', #20581, .T. ) ;
#16225=DIRECTION ( 'NONE',  ( -0.000000000000000000, -1.000000000000000000, -0.000000000000000000 ) ) ;
#16227=VECTOR ( 'NONE', #7779, 1000.000000000000000 ) ;
#16249=AXIS2_PLACEMENT_3D ( 'NONE', #24273, #28809, #21932 ) ;
#16258=EDGE_CURVE ( 'NONE', #2772, #27558, #4727, .T. ) ;
#16291=CIRCLE ( 'NONE', #7810, 11.99999999999998224 ) ;
#16292=CARTESIAN_POINT ( 'NONE',  ( -37.99999999999999289, 90.00000000000001421, -75.50000000000000000 ) ) ;
#16304=CARTESIAN_POINT ( 'NONE',  ( 37.99999999999999289, 90.00000000000001421, -75.50000000000001421 ) ) ;
#16325=AXIS2_PLACEMENT_3D ( 'NONE', #26115, #30632, #21435 ) ;
#16336=ADVANCED_FACE ( 'NONE', ( #9421 ), #14401, .F. ) ;
#16347=VECTOR ( 'NONE', #6287, 1000.000000000000000 ) ;
#16356=AXIS2_PLACEMENT_3D ( 'NONE', #8053, #10222, #10388 ) ;
#16414=DIRECTION ( 'NONE',  ( -1.000000000000000000, 0.000000000000000000, 0.000000000000000000 ) ) ;
#16418=ADVANCED_FACE ( 'NONE', ( #10336 ), #17512, .F. ) ;
#16426=DIRECTION ( 'NONE',  ( -0.000000000000000000, -0.000000000000000000, 1.000000000000000000 ) ) ;
#16429=ORIENTED_EDGE ( 'NONE', *, *, #23033, .T. ) ;
#16439=VECTOR ( 'NONE', #4088, 1000.000000000000000 ) ;
#16472=EDGE_CURVE ( 'NONE', #10292, #27407, #2552, .T. ) ;
#16484=DIRECTION ( 'NONE',  ( -0.000000000000000000, -0.000000000000000000, 1.000000000000000000 ) ) ;
#16500=LINE ( 'NONE', #28665, #159 ) ;
#16511=ORIENTED_EDGE ( 'NONE', *, *, #5276, .F. ) ;
#16525=FACE_OUTER_BOUND ( 'NONE', #6952, .T. ) ;
#16548=CARTESIAN_POINT ( 'NONE',  ( 4.851918296810534770, 49.76630973909864508, -40.79771880416375751 ) ) ;
#16550=DIRECTION ( 'NONE',  ( -1.000000000000000000, 0.000000000000000000, 0.000000000000000000 ) ) ;
#16562=DIRECTION ( 'NONE',  ( -1.000000000000000000, 0.000000000000000000, 0.000000000000000000 ) ) ;
#16568=VECTOR ( 'NONE', #7321, 1000.000000000000000 ) ;
#16570=DIRECTION ( 'NONE',  ( -0.000000000000000000, -0.000000000000000000, 1.000000000000000000 ) ) ;
#16705=ORIENTED_EDGE ( 'NONE', *, *, #9247, .T. ) ;
#16726=ORIENTED_EDGE ( 'NONE', *, *, #15458, .T. ) ;
#16804=ORIENTED_EDGE ( 'NONE', *, *, #14533, .F. ) ;
#16809=CARTESIAN_POINT ( 'NONE',  ( -9.906018991686922348, 49.01040375155087503, -43.72563556200963575 ) ) ;
#16818=LINE ( 'NONE', #19464, #18258 ) ;
#16838=ORIENTED_EDGE ( 'NONE', *, *, #28461, .F. ) ;
#16844=VERTEX_POINT ( 'NONE', #19350 ) ;
#16847=CARTESIAN_POINT ( 'NONE',  ( -70.00000000000000000, 70.00000000000000000, -92.50000000000000000 ) ) ;
#16863=VERTEX_POINT ( 'NONE', #22449 ) ;
#16868=LINE ( 'NONE', #7515, #20746 ) ;
#16961=ADVANCED_FACE ( 'NONE', ( #5626 ), #18092, .F. ) ;
#16978=CARTESIAN_POINT ( 'NONE',  ( 49.99999999999998579, -70.00000000000000000, -92.50000000000000000 ) ) ;
#16998=ORIENTED_EDGE ( 'NONE', *, *, #2320, .T. ) ;
#17003=EDGE_LOOP ( 'NONE', ( #23997, #25387, #607 ) ) ;
#17016=DIRECTION ( 'NONE',  ( -0.000000000000000000, -0.000000000000000000, 1.000000000000000000 ) ) ;
#17021=EDGE_LOOP ( 'NONE', ( #24593, #27463, #1315, #17279 ) ) ;
#17060=ADVANCED_FACE ( 'NONE', ( #21761 ), #28948, .F. ) ;
#17067=VECTOR ( 'NONE', #22616, 1000.000000000000000 ) ;
#17103=DIRECTION ( 'NONE',  ( -1.000000000000000000, 0.000000000000000000, 0.000000000000000000 ) ) ;
#17111=AXIS2_PLACEMENT_3D ( 'NONE', #16847, #9208, #9825 ) ;
#17113=CARTESIAN_POINT ( 'NONE',  ( -13.66229526048730669, 48.09760637535989503, -48.78872922615590824 ) ) ;
#17149=DIRECTION ( 'NONE',  ( 0.000000000000000000, 0.000000000000000000, -1.000000000000000000 ) ) ;
#17158=ORIENTED_EDGE ( 'NONE', *, *, #23783, .F. ) ;
#17160=CARTESIAN_POINT ( 'NONE',  ( 37.99999999999999289, 209.2686044187655909, -34.50000000000000000 ) ) ;
#17167=CYLINDRICAL_SURFACE ( 'NONE', #7848, 6.000000000000005329 ) ;
#17193=DIRECTION ( 'NONE',  ( -0.000000000000000000, 1.000000000000000000, -0.000000000000000000 ) ) ;
#17209=EDGE_LOOP ( 'NONE', ( #30392, #23592, #2625, #1480 ) ) ;
#17212=DIRECTION ( 'NONE',  ( 0.000000000000000000, -1.000000000000000000, 0.000000000000000000 ) ) ;
#17217=CARTESIAN_POINT ( 'NONE',  ( -37.99999999999999289, 70.00000000000000000, -22.50000000000001421 ) ) ;
#17233=SHAPE_DEFINITION_REPRESENTATION ( #24374, #20057 ) ;
#17260=CARTESIAN_POINT ( 'NONE',  ( 0.000000000000000000, 0.000000000000000000, -52.50000000000000000 ) ) ;
#17279=ORIENTED_EDGE ( 'NONE', *, *, #27114, .F. ) ;
#17381=PLANE ( 'NONE',  #28226 ) ;
#17386=FACE_OUTER_BOUND ( 'NONE', #4876, .T. ) ;
#17394=DIRECTION ( 'NONE',  ( -1.000000000000000000, 0.000000000000000000, 0.000000000000000000 ) ) ;
#17414=CARTESIAN_POINT ( 'NONE',  ( -57.50000000000001421, -50.00000000000000000, -87.50000000000000000 ) ) ;
#17436=EDGE_LOOP ( 'NONE', ( #460, #22643 ) ) ;
#17464=FACE_BOUND ( 'NONE', #21499, .T. ) ;
#17475=ORIENTED_EDGE ( 'NONE', *, *, #7671, .F. ) ;
#17486=DIRECTION ( 'NONE',  ( 0.000000000000000000, 1.000000000000000000, 0.000000000000000000 ) ) ;
#17512=PLANE ( 'NONE',  #26646 ) ;
#17514=ORIENTED_EDGE ( 'NONE', *, *, #8094, .T. ) ;
#17539=ORIENTED_EDGE ( 'NONE', *, *, #11841, .T. ) ;
#17566=EDGE_CURVE ( 'NONE', #4103, #26490, #18112, .T. ) ;
#17571=DIRECTION ( 'NONE',  ( 0.000000000000000000, 1.000000000000000000, 0.000000000000000000 ) ) ;
#17620=EDGE_CURVE ( 'NONE', #27015, #25122, #28693, .T. ) ;
#17622=ORIENTED_EDGE ( 'NONE', *, *, #24195, .F. ) ;
#17625=EDGE_LOOP ( 'NONE', ( #30404, #5429 ) ) ;
#17673=DIRECTION ( 'NONE',  ( -0.000000000000000000, 0.000000000000000000, 1.000000000000000000 ) ) ;
#17674=DIRECTION ( 'NONE',  ( 0.000000000000000000, 0.000000000000000000, -1.000000000000000000 ) ) ;
#17710=CYLINDRICAL_SURFACE ( 'NONE', #3839, 7.500000000000013323 ) ;
#17713=LINE ( 'NONE', #29896, #27283 ) ;
#17716=ORIENTED_EDGE ( 'NONE', *, *, #18492, .T. ) ;
#17719=STYLED_ITEM('',(#30879),#3175);
#17726=( NAMED_UNIT ( * ) SI_UNIT ( $, .STERADIAN. ) SOLID_ANGLE_UNIT ( ) );
#17730=EDGE_CURVE ( 'NONE', #11851, #11816, #2792, .T. ) ;
#17733=ADVANCED_FACE ( 'NONE', ( #10272 ), #19627, .F. ) ;
#17734=LINE ( 'NONE', #6040, #19264 ) ;
#17738=VERTEX_POINT ( 'NONE', #21974 ) ;
#17748=AXIS2_PLACEMENT_3D ( 'NONE', #22475, #10635, #13459 ) ;
#17774=CARTESIAN_POINT ( 'NONE',  ( -70.00000000000000000, 70.00000000000000000, -92.50000000000000000 ) ) ;
#17776=EDGE_CURVE ( 'NONE', #23138, #13113, #11205, .T. ) ;
#17784=DIRECTION ( 'NONE',  ( 0.000000000000000000, -1.000000000000000000, 0.000000000000000000 ) ) ;
#17788=CIRCLE ( 'NONE', #28240, 6.000000000000005329 ) ;
#17795=AXIS2_PLACEMENT_3D ( 'NONE', #2685, #7054, #16562 ) ;
#17799=ADVANCED_FACE ( 'NONE', ( #25702 ), #11978, .T. ) ;
#17830=EDGE_CURVE ( 'NONE', #16844, #9112, #27202, .T. ) ;
#17831=DIRECTION ( 'NONE',  ( 0.000000000000000000, 1.000000000000000000, 0.000000000000000000 ) ) ;
#17839=VECTOR ( 'NONE', #29719, 1000.000000000000000 ) ;
#17847=DIRECTION ( 'NONE',  ( 0.000000000000000000, 0.000000000000000000, 1.000000000000000000 ) ) ;
#17860=VERTEX_POINT ( 'NONE', #19599 ) ;
#17866=PLANE ( 'NONE',  #2647 ) ;
#17870=ORIENTED_EDGE ( 'NONE', *, *, #22020, .F. ) ;
#17902=ORIENTED_EDGE ( 'NONE', *, *, #26350, .T. ) ;
#17917=ORIENTED_EDGE ( 'NONE', *, *, #15654, .F. ) ;
#17921=DIRECTION ( 'NONE',  ( -1.000000000000000000, 0.000000000000000000, -0.000000000000000000 ) ) ;
#17961=DIRECTION ( 'NONE',  ( 0.000000000000000000, 0.000000000000000000, 1.000000000000000000 ) ) ;
#17972=DIRECTION ( 'NONE',  ( 1.000000000000000000, 0.000000000000000000, 0.000000000000000000 ) ) ;
#17996=CARTESIAN_POINT ( 'NONE',  ( 14.61451073016445967, 47.81658942982300431, -51.58549908343919554 ) ) ;
#18011=CARTESIAN_POINT ( 'NONE',  ( 49.99999999999997868, 90.00000000000001421, -34.50000000000000000 ) ) ;
#18021=DIRECTION ( 'NONE',  ( 1.000000000000000000, 0.000000000000000000, 0.000000000000000000 ) ) ;
#18039=CARTESIAN_POINT ( 'NONE',  ( -37.99999999999999289, 70.00000000000000000, -87.50000000000000000 ) ) ;
#18045=LINE ( 'NONE', #15688, #14445 ) ;
#18092=PLANE ( 'NONE',  #2249 ) ;
#18112=LINE ( 'NONE', #13450, #3803 ) ;
#18122=CARTESIAN_POINT ( 'NONE',  ( 32.50000000000000000, 3.980102097228898626E-15, -52.50000000000000000 ) ) ;
#18137=FACE_OUTER_BOUND ( 'NONE', #15506, .T. ) ;
#18139=VERTEX_POINT ( 'NONE', #26726 ) ;
#18147=CIRCLE ( 'NONE', #28092, 7.500000000000000000 ) ;
#18151=EDGE_CURVE ( 'NONE', #13747, #16188, #9293, .T. ) ;
#18195=ORIENTED_EDGE ( 'NONE', *, *, #3500, .T. ) ;
#18245=ORIENTED_EDGE ( 'NONE', *, *, #16472, .T. ) ;
#18258=VECTOR ( 'NONE', #582, 1000.000000000000000 ) ;
#18261=FACE_OUTER_BOUND ( 'NONE', #2888, .T. ) ;
#18274=DIRECTION ( 'NONE',  ( 0.000000000000000000, 1.000000000000000000, 0.000000000000000000 ) ) ;
#18304=AXIS2_PLACEMENT_3D ( 'NONE', #10392, #15363, #1187 ) ;
#18313=VECTOR ( 'NONE', #4205, 1000.000000000000000 ) ;
#18321=CLOSED_SHELL ( 'NONE', ( #1340, #26700, #18866, #7476, #22175, #9189, #11060, #14137, #8633, #17733, #17060, #9026, #22352, #27536, #19355, #13407, #16418, #16961, #29764, #7679, #9193, #15153, #6533, #20769, #9219, #16336, #3134, #30111, #3124, #9349, #1154, #480, #4395, #28489, #9163, #3841, #2100, #26804, #15439, #21173, #2745, #17799, #29752, #19929, #5391, #19122, #62, #2275, #14515, #27517, #13944, #15482, #11940, #10353, #12107, #1766, #15491, #5028, #1091, #28272 ) ) ;
#18326=AXIS2_PLACEMENT_3D ( 'NONE', #7032, #25465, #4090 ) ;
#18332=EDGE_CURVE ( 'NONE', #10292, #21897, #15412, .T. ) ;
#18342=ORIENTED_EDGE ( 'NONE', *, *, #5764, .F. ) ;
#18365=AXIS2_PLACEMENT_3D ( 'NONE', #26261, #23921, #21260 ) ;
#18379=ORIENTED_EDGE ( 'NONE', *, *, #7257, .T. ) ;
#18414=AXIS2_PLACEMENT_3D ( 'NONE', #23319, #1960, #9129 ) ;
#18439=DIRECTION ( 'NONE',  ( 0.000000000000000000, 0.000000000000000000, -1.000000000000000000 ) ) ;
#18440=CARTESIAN_POINT ( 'NONE',  ( 49.99999999999998579, 50.00000000000000000, -87.50000000000000000 ) ) ;
#18444=CARTESIAN_POINT ( 'NONE',  ( 49.99999999999998579, 50.00000000000000000, -92.50000000000000000 ) ) ;
#18468=ORIENTED_EDGE ( 'NONE', *, *, #4048, .F. ) ;
#18482=DIRECTION ( 'NONE',  ( 0.000000000000000000, 0.000000000000000000, -1.000000000000000000 ) ) ;
#18492=EDGE_CURVE ( 'NONE', #9106, #13113, #16868, .T. ) ;
#18500=DIRECTION ( 'NONE',  ( -1.000000000000000000, 0.000000000000000000, 0.000000000000000000 ) ) ;
#18540=CIRCLE ( 'NONE', #22504, 7.500000000000000000 ) ;
#18546=DIRECTION ( 'NONE',  ( 0.000000000000000000, 0.000000000000000000, -1.000000000000000000 ) ) ;
#18547=EDGE_LOOP ( 'NONE', ( #16705, #16511, #18342, #19873 ) ) ;
#18566=VECTOR ( 'NONE', #26125, 1000.000000000000000 ) ;
#18581=CARTESIAN_POINT ( 'NONE',  ( 32.50000000000000000, 3.980102097228898626E-15, -52.50000000000000000 ) ) ;
#18588=EDGE_CURVE ( 'NONE', #27029, #24252, #10544, .T. ) ;
#18599=VERTEX_POINT ( 'NONE', #24725 ) ;
#18608=AXIS2_PLACEMENT_3D ( 'NONE', #19703, #12861, #17847 ) ;
#18632=ORIENTED_EDGE ( 'NONE', *, *, #8434, .T. ) ;
#18646=CARTESIAN_POINT ( 'NONE',  ( 49.99999999999998579, 50.00000000000000000, 12.49999999999998401 ) ) ;
#18680=DIRECTION ( 'NONE',  ( 1.000000000000000000, 0.000000000000000000, 0.000000000000000000 ) ) ;
#18697=ORIENTED_EDGE ( 'NONE', *, *, #1489, .T. ) ;
#18698=ORIENTED_EDGE ( 'NONE', *, *, #30363, .F. ) ;
#18703=CIRCLE ( 'NONE', #11732, 6.000000000000005329 ) ;
#18704=ORIENTED_EDGE ( 'NONE', *, *, #17566, .T. ) ;
#18719=ORIENTED_EDGE ( 'NONE', *, *, #12618, .F. ) ;
#18781=DIRECTION ( 'NONE',  ( 1.000000000000000000, 0.000000000000000000, 0.000000000000000000 ) ) ;
#18809=ORIENTED_EDGE ( 'NONE', *, *, #22020, .T. ) ;
#18848=ORIENTED_EDGE ( 'NONE', *, *, #757, .F. ) ;
#18850=DIRECTION ( 'NONE',  ( 0.000000000000000000, 0.000000000000000000, 1.000000000000000000 ) ) ;
#18853=AXIS2_PLACEMENT_3D ( 'NONE', #30470, #11463, #27849 ) ;
#18863=AXIS2_PLACEMENT_3D ( 'NONE', #11518, #9167, #18680 ) ;
#18866=ADVANCED_FACE ( 'NONE', ( #13196 ), #6626, .F. ) ;
#18871=LINE ( 'NONE', #16978, #3586 ) ;
#18887=LINE ( 'NONE', #28398, #14322 ) ;
#18902=AXIS2_PLACEMENT_3D ( 'NONE', #7355, #24167, #22149 ) ;
#18908=EDGE_CURVE ( 'NONE', #27029, #26519, #6815, .T. ) ;
#18914=CARTESIAN_POINT ( 'NONE',  ( 69.99999999999998579, -50.00000000000000000, -92.50000000000000000 ) ) ;
#18915=ORIENTED_EDGE ( 'NONE', *, *, #28094, .T. ) ;
#18916=EDGE_CURVE ( 'NONE', #16863, #2233, #17788, .T. ) ;
#18920=EDGE_LOOP ( 'NONE', ( #23267, #23963 ) ) ;
#18951=ORIENTED_EDGE ( 'NONE', *, *, #27142, .T. ) ;
#18954=DIRECTION ( 'NONE',  ( -0.000000000000000000, -0.000000000000000000, -1.000000000000000000 ) ) ;
#18957=ORIENTED_EDGE ( 'NONE', *, *, #22370, .T. ) ;
#18959=CYLINDRICAL_SURFACE ( 'NONE', #16325, 6.000000000000005329 ) ;
#18995=LINE ( 'NONE', #6984, #15885 ) ;
#18997=DIRECTION ( 'NONE',  ( 0.000000000000000000, 0.000000000000000000, -1.000000000000000000 ) ) ;
#19041=CARTESIAN_POINT ( 'NONE',  ( -37.99999999999999289, 70.00000000000000000, -75.50000000000000000 ) ) ;
#19043=DIRECTION ( 'NONE',  ( 0.000000000000000000, 0.000000000000000000, 1.000000000000000000 ) ) ;
#19049=CARTESIAN_POINT ( 'NONE',  ( 9.149370483914699648, 49.15727498498932135, -43.10339609117139759 ) ) ;
#19071=AXIS2_PLACEMENT_3D ( 'NONE', #22210, #12712, #845 ) ;
#19072=ORIENTED_EDGE ( 'NONE', *, *, #18151, .F. ) ;
#19076=DIRECTION ( 'NONE',  ( 0.000000000000000000, 0.000000000000000000, -1.000000000000000000 ) ) ;
#19100=DIRECTION ( 'NONE',  ( -0.000000000000000000, 0.000000000000000000, 1.000000000000000000 ) ) ;
#19114=EDGE_LOOP ( 'NONE', ( #7960, #12635, #10295, #2725 ) ) ;
#19122=ADVANCED_FACE ( 'NONE', ( #12763 ), #10578, .F. ) ;
#19151=CARTESIAN_POINT ( 'NONE',  ( -11.90245152369472059, 48.56370570873113479, -64.14171519351066308 ) ) ;
#19156=ORIENTED_EDGE ( 'NONE', *, *, #11667, .F. ) ;
#19163=EDGE_LOOP ( 'NONE', ( #18957, #18245, #29783, #15010 ) ) ;
#19164=CARTESIAN_POINT ( 'NONE',  ( 37.99999999999999289, 90.00000000000001421, -40.50000000000000711 ) ) ;
#19185=LINE ( 'NONE', #5467, #10250 ) ;
#19192=CYLINDRICAL_SURFACE ( 'NONE', #11396, 6.000000000000005329 ) ;
#19219=CYLINDRICAL_SURFACE ( 'NONE', #22655, 50.00000000000000000 ) ;
#19264=VECTOR ( 'NONE', #15550, 1000.000000000000000 ) ;
#19295=EDGE_CURVE ( 'NONE', #22222, #29647, #25771, .T. ) ;
#19305=CARTESIAN_POINT ( 'NONE',  ( -9.148437479020795848, 49.15745090874974466, -43.10266427149625201 ) ) ;
#19330=DIRECTION ( 'NONE',  ( 0.000000000000000000, 1.000000000000000000, 0.000000000000000000 ) ) ;
#19338=FACE_OUTER_BOUND ( 'NONE', #4578, .T. ) ;
#19344=CIRCLE ( 'NONE', #11388, 7.500000000000000000 ) ;
#19349=CIRCLE ( 'NONE', #5905, 6.000000000000005329 ) ;
#19350=CARTESIAN_POINT ( 'NONE',  ( 37.99999999999999289, 70.00000000000000000, -81.50000000000001421 ) ) ;
#19355=ADVANCED_FACE ( 'NONE', ( #6362 ), #13694, .F. ) ;
#19363=CARTESIAN_POINT ( 'NONE',  ( 37.99999999999999289, 209.2686044187655909, -34.50000000000000000 ) ) ;
#19443=CIRCLE ( 'NONE', #9964, 11.99999999999999645 ) ;
#19455=CARTESIAN_POINT ( 'NONE',  ( -7.531728742324322212, 49.43635587137926990, -41.99112863159430020 ) ) ;
#19461=ORIENTED_EDGE ( 'NONE', *, *, #1965, .T. ) ;
#19464=CARTESIAN_POINT ( 'NONE',  ( 69.99999999999998579, -70.00000000000000000, -92.50000000000000000 ) ) ;
#19514=CARTESIAN_POINT ( 'NONE',  ( 0.000000000000000000, 0.000000000000000000, -52.50000000000000000 ) ) ;
#19528=EDGE_CURVE ( 'NONE', #28201, #15417, #10390, .T. ) ;
#19543=CARTESIAN_POINT ( 'NONE',  ( -50.00000000000000000, 0.000000000000000000, -87.50000000000000000 ) ) ;
#19548=CARTESIAN_POINT ( 'NONE',  ( 12.50000000000000000, 1.530808498934191521E-15, -52.50000000000000000 ) ) ;
#19568=EDGE_LOOP ( 'NONE', ( #21942, #21357, #24181, #9652 ) ) ;
#19599=CARTESIAN_POINT ( 'NONE',  ( 49.99999999999998579, -70.00000000000000000, 12.49999999999999112 ) ) ;
#19606=CARTESIAN_POINT ( 'NONE',  ( -14.03716236476662615, 47.98954181453471080, -49.68998407197084788 ) ) ;
#19615=VERTEX_POINT ( 'NONE', #17414 ) ;
#19627=CYLINDRICAL_SURFACE ( 'NONE', #3306, 7.500000000000013323 ) ;
#19645=ORIENTED_EDGE ( 'NONE', *, *, #11667, .T. ) ;
#19676=EDGE_CURVE ( 'NONE', #4103, #27029, #20508, .T. ) ;
#19701=PLANE ( 'NONE',  #2635 ) ;
#19703=CARTESIAN_POINT ( 'NONE',  ( 37.99999999999999289, 70.00000000000000000, -34.50000000000000000 ) ) ;
#19713=AXIS2_PLACEMENT_3D ( 'NONE', #6412, #29821, #30263 ) ;
#19715=ORIENTED_EDGE ( 'NONE', *, *, #3679, .F. ) ;
#19720=DIRECTION ( 'NONE',  ( -1.000000000000000000, -0.000000000000000000, -0.000000000000000000 ) ) ;
#19747=DIRECTION ( 'NONE',  ( -0.000000000000000000, -0.000000000000000000, -1.000000000000000000 ) ) ;
#19755=CARTESIAN_POINT ( 'NONE',  ( -3.420703685013330553, 49.88518064725936796, -40.38700250513966239 ) ) ;
#19772=AXIS2_PLACEMENT_3D ( 'NONE', #14089, #25961, #30788 ) ;
#19781=ORIENTED_EDGE ( 'NONE', *, *, #3850, .T. ) ;
#19805=EDGE_CURVE ( 'NONE', #20793, #4103, #14263, .T. ) ;
#19815=AXIS2_PLACEMENT_3D ( 'NONE', #18646, #9444, #18500 ) ;
#19845=ORIENTED_EDGE ( 'NONE', *, *, #20427, .T. ) ;
#19847=CIRCLE ( 'NONE', #16356, 11.99999999999998934 ) ;
#19873=ORIENTED_EDGE ( 'NONE', *, *, #7813, .T. ) ;
#19899=FACE_OUTER_BOUND ( 'NONE', #23651, .T. ) ;
#19913=DIRECTION ( 'NONE',  ( 0.000000000000000000, 0.000000000000000000, -1.000000000000000000 ) ) ;
#19929=ADVANCED_FACE ( 'NONE', ( #12700 ), #15166, .T. ) ;
#19938=CYLINDRICAL_SURFACE ( 'NONE', #12352, 11.99999999999998934 ) ;
#19944=CARTESIAN_POINT ( 'NONE',  ( 42.49999999999998579, -50.00000000000000000, 12.49999999999999112 ) ) ;
#19953=CARTESIAN_POINT ( 'NONE',  ( 0.000000000000000000, 0.000000000000000000, -87.50000000000000000 ) ) ;
#19955=EDGE_LOOP ( 'NONE', ( #12607, #4094 ) ) ;
#19970=ORIENTED_EDGE ( 'NONE', *, *, #12618, .T. ) ;
#20009=DIRECTION ( 'NONE',  ( 0.000000000000000000, 1.000000000000000000, -0.000000000000000000 ) ) ;
#20012=CARTESIAN_POINT ( 'NONE',  ( 37.99999999999999289, 209.2686044187655909, -75.50000000000001421 ) ) ;
#20034=FACE_OUTER_BOUND ( 'NONE', #2935, .T. ) ;
#20057=SHAPE_REPRESENTATION ( 'Housing End Cover Cap', ( #7396 ), #9395 ) ;
#20071=CARTESIAN_POINT ( 'NONE',  ( -3.915634928944694781, 49.85588857687934450, -69.51358094991340408 ) ) ;
#20105=DIRECTION ( 'NONE',  ( 0.000000000000000000, 1.000000000000000000, 0.000000000000000000 ) ) ;
#20138=DIRECTION ( 'NONE',  ( 0.000000000000000000, 0.000000000000000000, 1.000000000000000000 ) ) ;
#20143=CIRCLE ( 'NONE', #14161, 6.000000000000005329 ) ;
#20162=CARTESIAN_POINT ( 'NONE',  ( 14.90335466576768120, 47.72767136615566130, -53.03506201841181422 ) ) ;
#20181=ORIENTED_EDGE ( 'NONE', *, *, #27680, .F. ) ;
#20182=CARTESIAN_POINT ( 'NONE',  ( -70.00000000000000000, 70.00000000000000000, -92.50000000000000000 ) ) ;
#20216=FACE_OUTER_BOUND ( 'NONE', #1529, .T. ) ;
#20217=CARTESIAN_POINT ( 'NONE',  ( -32.50000000000000000, 0.000000000000000000, -87.50000000000000000 ) ) ;
#20219=SHAPE_REPRESENTATION_RELATIONSHIP ( 'NONE' , 'NONE' ,  #20057, #9148 ) ;
#20236=AXIS2_PLACEMENT_3D ( 'NONE', #6981, #9476, #9313 ) ;
#20243=LINE ( 'NONE', #22429, #23086 ) ;
#20285=ORIENTED_EDGE ( 'NONE', *, *, #5216, .T. ) ;
#20302=CARTESIAN_POINT ( 'NONE',  ( 49.99999999999998579, 50.00000000000000000, -92.50000000000000000 ) ) ;
#20310=CIRCLE ( 'NONE', #27801, 11.99999999999998934 ) ;
#20326=CARTESIAN_POINT ( 'NONE',  ( 14.03875201089029190, 47.98907823057331257, -49.69408436906743987 ) ) ;
#20356=VECTOR ( 'NONE', #3885, 1000.000000000000000 ) ;
#20367=DIRECTION ( 'NONE',  ( 0.000000000000000000, 0.000000000000000000, -1.000000000000000000 ) ) ;
#20372=CARTESIAN_POINT ( 'NONE',  ( -50.00000000000000000, 70.00000000000000000, 12.49999999999999112 ) ) ;
#20373=DIRECTION ( 'NONE',  ( 0.000000000000000000, -0.000000000000000000, 1.000000000000000000 ) ) ;
#20390=VERTEX_POINT ( 'NONE', #10418 ) ;
#20399=VERTEX_POINT ( 'NONE', #15078 ) ;
#20427=EDGE_CURVE ( 'NONE', #15471, #16863, #17734, .T. ) ;
#20450=DIRECTION ( 'NONE',  ( 0.000000000000000000, 1.000000000000000000, 0.000000000000000000 ) ) ;
#20460=FACE_BOUND ( 'NONE', #18920, .T. ) ;
#20475=CARTESIAN_POINT ( 'NONE',  ( 10.26717756958418981, 48.93576106897143774, -44.05370344458894039 ) ) ;
#20505=DIRECTION ( 'NONE',  ( 0.000000000000000000, 0.000000000000000000, -1.000000000000000000 ) ) ;
#20508=LINE ( 'NONE', #30178, #30293 ) ;
#20516=LINE ( 'NONE', #30038, #14825 ) ;
#20553=LINE ( 'NONE', #25238, #20356 ) ;
#20565=EDGE_LOOP ( 'NONE', ( #17716, #28096, #14207, #18379, #10983, #12377, #3737, #23293 ) ) ;
#20579=CARTESIAN_POINT ( 'NONE',  ( 49.99999999999998579, 90.00000000000001421, -75.50000000000001421 ) ) ;
#20581=EDGE_LOOP ( 'NONE', ( #10028, #19845, #22482, #7767 ) ) ;
#20636=EDGE_CURVE ( 'NONE', #15437, #27015, #23235, .T. ) ;
#20651=CARTESIAN_POINT ( 'NONE',  ( 49.99999999999998579, 70.00000000000000000, -75.50000000000001421 ) ) ;
#20656=EDGE_CURVE ( 'NONE', #21977, #3976, #2835, .T. ) ;
#20660=DIRECTION ( 'NONE',  ( 0.000000000000000000, 0.000000000000000000, 1.000000000000000000 ) ) ;
#20711=DIRECTION ( 'NONE',  ( 0.000000000000000000, 1.000000000000000000, 0.000000000000000000 ) ) ;
#20715=VECTOR ( 'NONE', #878, 1000.000000000000000 ) ;
#20731=FACE_OUTER_BOUND ( 'NONE', #17209, .T. ) ;
#20738=FACE_OUTER_BOUND ( 'NONE', #15870, .T. ) ;
#20746=VECTOR ( 'NONE', #17486, 1000.000000000000000 ) ;
#20748=DIRECTION ( 'NONE',  ( 0.000000000000000000, 0.000000000000000000, 1.000000000000000000 ) ) ;
#20755=CARTESIAN_POINT ( 'NONE',  ( -37.99999999999999289, 90.00000000000001421, -87.50000000000000000 ) ) ;
#20764=DIRECTION ( 'NONE',  ( 0.000000000000000000, 0.000000000000000000, -1.000000000000000000 ) ) ;
#20769=ADVANCED_FACE ( 'NONE', ( #2043 ), #2349, .T. ) ;
#20774=CIRCLE ( 'NONE', #18304, 12.50000000000000000 ) ;
#20793=VERTEX_POINT ( 'NONE', #20755 ) ;
#20799=VERTEX_POINT ( 'NONE', #1897 ) ;
#20809=EDGE_CURVE ( 'NONE', #10117, #15581, #4538, .T. ) ;
#20824=PLANE ( 'NONE',  #18414 ) ;
#20837=AXIS2_PLACEMENT_3D ( 'NONE', #17260, #19747, #28963 ) ;
#20860=DIRECTION ( 'NONE',  ( -0.000000000000000000, -0.000000000000000000, -1.000000000000000000 ) ) ;
#20883=ORIENTED_EDGE ( 'NONE', *, *, #8308, .F. ) ;
#20900=DIRECTION ( 'NONE',  ( 0.000000000000000000, 0.000000000000000000, -1.000000000000000000 ) ) ;
#20903=DIRECTION ( 'NONE',  ( 0.000000000000000000, 0.000000000000000000, -1.000000000000000000 ) ) ;
#20921=CIRCLE ( 'NONE', #4994, 12.50000000000000000 ) ;
#20923=DIRECTION ( 'NONE',  ( 0.000000000000000000, 0.000000000000000000, -1.000000000000000000 ) ) ;
#20967=EDGE_LOOP ( 'NONE', ( #616, #18704, #227, #30757 ) ) ;
#21010=ORIENTED_EDGE ( 'NONE', *, *, #22370, .F. ) ;
#21014=DIRECTION ( 'NONE',  ( 1.000000000000000000, 0.000000000000000000, 0.000000000000000000 ) ) ;
#21023=VERTEX_POINT ( 'NONE', #25878 ) ;
#21048=LINE ( 'NONE', #18581, #30278 ) ;
#21052=ORIENTED_EDGE ( 'NONE', *, *, #16213, .F. ) ;
#21061=CIRCLE ( 'NONE', #24544, 6.000000000000005329 ) ;
#21075=LINE ( 'NONE', #9238, #16347 ) ;
#21083=LINE ( 'NONE', #9553, #10100 ) ;
#21086=DIRECTION ( 'NONE',  ( -1.000000000000000000, 0.000000000000000000, 0.000000000000000000 ) ) ;
#21091=DIRECTION ( 'NONE',  ( -1.000000000000000000, 0.000000000000000000, 0.000000000000000000 ) ) ;
#21116=DIRECTION ( 'NONE',  ( -0.000000000000000000, -1.000000000000000000, -0.000000000000000000 ) ) ;
#21173=ADVANCED_FACE ( 'NONE', ( #29138 ), #19938, .T. ) ;
#21188=PLANE ( 'NONE',  #7834 ) ;
#21205=ORIENTED_EDGE ( 'NONE', *, *, #28277, .T. ) ;
#21208=AXIS2_PLACEMENT_3D ( 'NONE', #7223, #30057, #18781 ) ;
#21260=DIRECTION ( 'NONE',  ( -1.000000000000000000, 0.000000000000000000, 0.000000000000000000 ) ) ;
#21263=CIRCLE ( 'NONE', #14296, 6.000000000000005329 ) ;
#21325=VECTOR ( 'NONE', #29377, 1000.000000000000000 ) ;
#21357=ORIENTED_EDGE ( 'NONE', *, *, #25163, .T. ) ;
#21376=EDGE_LOOP ( 'NONE', ( #13720, #14034, #18848, #26289 ) ) ;
#21413=ORIENTED_EDGE ( 'NONE', *, *, #30153, .F. ) ;
#21435=DIRECTION ( 'NONE',  ( 0.000000000000000000, 0.000000000000000000, -1.000000000000000000 ) ) ;
#21439=CARTESIAN_POINT ( 'NONE',  ( -37.99999999999999289, 90.00000000000001421, -34.49999999999999289 ) ) ;
#21469=CARTESIAN_POINT ( 'NONE',  ( 37.99999999999999289, 90.00000000000001421, -75.50000000000001421 ) ) ;
#21476=CARTESIAN_POINT ( 'NONE',  ( -70.00000000000000000, 70.00000000000000000, -92.50000000000000000 ) ) ;
#21482=ORIENTED_EDGE ( 'NONE', *, *, #23869, .F. ) ;
#21499=EDGE_LOOP ( 'NONE', ( #5370, #27031 ) ) ;
#21578=AXIS2_PLACEMENT_3D ( 'NONE', #2295, #18546, #28046 ) ;
#21606=VECTOR ( 'NONE', #19720, 1000.000000000000000 ) ;
#21656=CYLINDRICAL_SURFACE ( 'NONE', #30786, 12.50000000000000000 ) ;
#21660=DIRECTION ( 'NONE',  ( -1.000000000000000000, 0.000000000000000000, 0.000000000000000000 ) ) ;
#21702=VECTOR ( 'NONE', #2641, 1000.000000000000000 ) ;
#21742=CYLINDRICAL_SURFACE ( 'NONE', #19071, 20.00000000000000000 ) ;
#21760=AXIS2_PLACEMENT_3D ( 'NONE', #29187, #27017, #20138 ) ;
#21761=FACE_OUTER_BOUND ( 'NONE', #7345, .T. ) ;
#21785=EDGE_CURVE ( 'NONE', #24252, #8036, #19847, .T. ) ;
#21793=CARTESIAN_POINT ( 'NONE',  ( -11.29794076498435551, 48.71192074315335674, -45.08525989437928416 ) ) ;
#21813=EDGE_CURVE ( 'NONE', #10182, #22039, #3985, .T. ) ;
#21826=ORIENTED_EDGE ( 'NONE', *, *, #14533, .T. ) ;
#21872=CARTESIAN_POINT ( 'NONE',  ( 37.99999999999999289, 209.2686044187655909, -28.49999999999999645 ) ) ;
#21897=VERTEX_POINT ( 'NONE', #9113 ) ;
#21905=ORIENTED_EDGE ( 'NONE', *, *, #20427, .F. ) ;
#21921=ORIENTED_EDGE ( 'NONE', *, *, #1489, .F. ) ;
#21926=EDGE_CURVE ( 'NONE', #3976, #21977, #12373, .T. ) ;
#21932=DIRECTION ( 'NONE',  ( 1.000000000000000000, 0.000000000000000000, 0.000000000000000000 ) ) ;
#21942=ORIENTED_EDGE ( 'NONE', *, *, #5558, .F. ) ;
#21945=CARTESIAN_POINT ( 'NONE',  ( -14.97621673923063312, 47.70446069948408763, -55.98035886673119421 ) ) ;
#21961=ORIENTED_EDGE ( 'NONE', *, *, #14370, .F. ) ;
#21974=CARTESIAN_POINT ( 'NONE',  ( 69.99999999999998579, -50.00000000000000000, 12.49999999999999112 ) ) ;
#21977=VERTEX_POINT ( 'NONE', #7853 ) ;
#21985=EDGE_CURVE ( 'NONE', #9360, #20390, #22189, .T. ) ;
#22014=DIRECTION ( 'NONE',  ( 0.000000000000000000, 1.000000000000000000, 0.000000000000000000 ) ) ;
#22020=EDGE_CURVE ( 'NONE', #27558, #22434, #8322, .T. ) ;
#22025=DIRECTION ( 'NONE',  ( 0.000000000000000000, 0.000000000000000000, -1.000000000000000000 ) ) ;
#22039=VERTEX_POINT ( 'NONE', #3320 ) ;
#22063=DIRECTION ( 'NONE',  ( 0.000000000000000000, 0.000000000000000000, 1.000000000000000000 ) ) ;
#22078=( NAMED_UNIT ( * ) PLANE_ANGLE_UNIT ( ) SI_UNIT ( $, .RADIAN. ) );
#22094=CIRCLE ( 'NONE', #182, 20.00000000000000355 ) ;
#22124=FACE_BOUND ( 'NONE', #3266, .T. ) ;
#22149=DIRECTION ( 'NONE',  ( -1.000000000000000000, 0.000000000000000000, 0.000000000000000000 ) ) ;
#22175=ADVANCED_FACE ( 'NONE', ( #4268 ), #19192, .F. ) ;
#22189=LINE ( 'NONE', #19548, #25819 ) ;
#22197=CARTESIAN_POINT ( 'NONE',  ( -70.00000000000000000, 70.00000000000000000, -92.50000000000000000 ) ) ;
#22210=CARTESIAN_POINT ( 'NONE',  ( -50.00000000000000000, -50.00000000000000000, -92.50000000000000000 ) ) ;
#22216=CARTESIAN_POINT ( 'NONE',  ( 69.99999999999998579, -70.00000000000000000, -92.50000000000000000 ) ) ;
#22222=VERTEX_POINT ( 'NONE', #22611 ) ;
#22231=VECTOR ( 'NONE', #5663, 1000.000000000000000 ) ;
#22252=CARTESIAN_POINT ( 'NONE',  ( 1.837104849652355830E-15, 50.00000000000000000, -70.00000000000000000 ) ) ;
#22281=DIRECTION ( 'NONE',  ( 0.000000000000000000, -0.4961389383568337030, 0.8682431421244592995 ) ) ;
#22291=DIRECTION ( 'NONE',  ( 0.000000000000000000, -1.000000000000000000, 0.000000000000000000 ) ) ;
#22303=AXIS2_PLACEMENT_3D ( 'NONE', #24358, #3004, #12522 ) ;
#22310=DIRECTION ( 'NONE',  ( -1.000000000000000000, 0.000000000000000000, 0.000000000000000000 ) ) ;
#22311=DIRECTION ( 'NONE',  ( 0.000000000000000000, 0.000000000000000000, -1.000000000000000000 ) ) ;
#22333=VECTOR ( 'NONE', #18954, 1000.000000000000000 ) ;
#22352=ADVANCED_FACE ( 'NONE', ( #7762 ), #432, .F. ) ;
#22368=LINE ( 'NONE', #27371, #13082 ) ;
#22370=EDGE_CURVE ( 'NONE', #21897, #10292, #11830, .T. ) ;
#22411=CARTESIAN_POINT ( 'NONE',  ( -7.523478279969216587, 49.43269233655315276, -67.98621439856492543 ) ) ;
#22429=CARTESIAN_POINT ( 'NONE',  ( -70.00000000000000000, 70.00000000000000000, 12.49999999999999112 ) ) ;
#22434=VERTEX_POINT ( 'NONE', #20217 ) ;
#22444=FACE_OUTER_BOUND ( 'NONE', #24104, .T. ) ;
#22445=PLANE ( 'NONE',  #26628 ) ;
#22449=CARTESIAN_POINT ( 'NONE',  ( -37.99999999999999289, 70.00000000000000000, -69.49999999999998579 ) ) ;
#22475=CARTESIAN_POINT ( 'NONE',  ( -49.99999999999998579, 209.2686044187655909, -75.50000000000002842 ) ) ;
#22482=ORIENTED_EDGE ( 'NONE', *, *, #29793, .F. ) ;
#22484=DIRECTION ( 'NONE',  ( 1.000000000000000000, 0.000000000000000000, 0.000000000000000000 ) ) ;
#22486=ORIENTED_EDGE ( 'NONE', *, *, #30503, .F. ) ;
#22492=CARTESIAN_POINT ( 'NONE',  ( 4.852933661107258878, 49.77225640444542876, -69.22700773620653081 ) ) ;
#22504=AXIS2_PLACEMENT_3D ( 'NONE', #8559, #28175, #6806 ) ;
#22560=EDGE_CURVE ( 'NONE', #8734, #2233, #6792, .T. ) ;
#22562=AXIS2_PLACEMENT_3D ( 'NONE', #13319, #20923, #25316 ) ;
#22571=EDGE_LOOP ( 'NONE', ( #4752, #28348, #26567, #16838, #1101 ) ) ;
#22597=LINE ( 'NONE', #10603, #29524 ) ;
#22601=DIRECTION ( 'NONE',  ( 0.000000000000000000, -1.000000000000000000, 0.000000000000000000 ) ) ;
#22611=CARTESIAN_POINT ( 'NONE',  ( -57.50000000000001421, 50.00000000000000000, 12.49999999999999112 ) ) ;
#22616=DIRECTION ( 'NONE',  ( 0.000000000000000000, 0.000000000000000000, -1.000000000000000000 ) ) ;
#22643=ORIENTED_EDGE ( 'NONE', *, *, #15654, .T. ) ;
#22646=CARTESIAN_POINT ( 'NONE',  ( 7.944760815330115911, 49.36648745528790982, -67.73260676410613712 ) ) ;
#22655=AXIS2_PLACEMENT_3D ( 'NONE', #26881, #3011, #5502 ) ;
#22686=FACE_OUTER_BOUND ( 'NONE', #11782, .T. ) ;
#22711=EDGE_LOOP ( 'NONE', ( #1353, #25851, #7737, #17917 ) ) ;
#22785=ORIENTED_EDGE ( 'NONE', *, *, #2320, .F. ) ;
#22813=CARTESIAN_POINT ( 'NONE',  ( 15.00007558036415567, 47.69693630192244882, -54.01249125054359723 ) ) ;
#22817=CARTESIAN_POINT ( 'NONE',  ( 37.99999999999999289, 70.00000000000000000, -87.50000000000000000 ) ) ;
#22846=ORIENTED_EDGE ( 'NONE', *, *, #19805, .F. ) ;
#22863=VERTEX_POINT ( 'NONE', #14729 ) ;
#22899=ORIENTED_EDGE ( 'NONE', *, *, #24204, .T. ) ;
#22919=EDGE_CURVE ( 'NONE', #21897, #6185, #5499, .T. ) ;
#22955=CIRCLE ( 'NONE', #24965, 7.500000000000013323 ) ;
#23033=EDGE_CURVE ( 'NONE', #9360, #25532, #26874, .T. ) ;
#23041=ORIENTED_EDGE ( 'NONE', *, *, #25163, .F. ) ;
#23069=DIRECTION ( 'NONE',  ( -1.000000000000000000, 0.000000000000000000, 0.000000000000000000 ) ) ;
#23086=VECTOR ( 'NONE', #30479, 1000.000000000000000 ) ;
#23106=CARTESIAN_POINT ( 'NONE',  ( 0.9819813860070594203, 49.99276302178526521, -69.97593018308113244 ) ) ;
#23138=VERTEX_POINT ( 'NONE', #29161 ) ;
#23175=ORIENTED_EDGE ( 'NONE', *, *, #9642, .F. ) ;
#23204=VECTOR ( 'NONE', #28960, 1000.000000000000000 ) ;
#23212=ORIENTED_EDGE ( 'NONE', *, *, #15462, .F. ) ;
#23215=AXIS2_PLACEMENT_3D ( 'NONE', #23640, #2282, #11804 ) ;
#23222=ORIENTED_EDGE ( 'NONE', *, *, #30716, .T. ) ;
#23231=CYLINDRICAL_SURFACE ( 'NONE', #12809, 6.000000000000005329 ) ;
#23235=CIRCLE ( 'NONE', #27242, 6.000000000000005329 ) ;
#23246=DIRECTION ( 'NONE',  ( -1.000000000000000000, 0.000000000000000000, 0.000000000000000000 ) ) ;
#23267=ORIENTED_EDGE ( 'NONE', *, *, #12144, .F. ) ;
#23279=DIRECTION ( 'NONE',  ( 0.000000000000000000, 0.000000000000000000, -1.000000000000000000 ) ) ;
#23293=ORIENTED_EDGE ( 'NONE', *, *, #7815, .T. ) ;
#23319=CARTESIAN_POINT ( 'NONE',  ( 49.99999999999998579, 209.2686044187655909, -75.50000000000001421 ) ) ;
#23347=PRODUCT_DEFINITION_FORMATION_WITH_SPECIFIED_SOURCE ( 'ANY', '', #4943, .NOT_KNOWN. ) ;
#23351=CARTESIAN_POINT ( 'NONE',  ( 35.00000000000000000, 90.00000000000001421, -22.50000000000002487 ) ) ;
#23352=AXIS2_PLACEMENT_3D ( 'NONE', #10275, #8682, #20373 ) ;
#23392=ORIENTED_EDGE ( 'NONE', *, *, #18332, .F. ) ;
#23441=VERTEX_POINT ( 'NONE', #8802 ) ;
#23477=EDGE_CURVE ( 'NONE', #946, #8162, #7474, .T. ) ;
#23531=ORIENTED_EDGE ( 'NONE', *, *, #26915, .T. ) ;
#23548=CARTESIAN_POINT ( 'NONE',  ( 49.99999999999998579, 209.2686044187655909, -75.50000000000001421 ) ) ;
#23592=ORIENTED_EDGE ( 'NONE', *, *, #30503, .T. ) ;
#23636=AXIS2_PLACEMENT_3D ( 'NONE', #30166, #27677, #18021 ) ;
#23640=CARTESIAN_POINT ( 'NONE',  ( 0.000000000000000000, 0.000000000000000000, -52.50000000000000000 ) ) ;
#23651=EDGE_LOOP ( 'NONE', ( #17475, #7415, #29526, #24633 ) ) ;
#23705=CIRCLE ( 'NONE', #10271, 20.00000000000000355 ) ;
#23728=CYLINDRICAL_SURFACE ( 'NONE', #17795, 7.500000000000000000 ) ;
#23736=CARTESIAN_POINT ( 'NONE',  ( 69.99999999999998579, 70.00000000000000000, 12.49999999999999112 ) ) ;
#23754=VERTEX_POINT ( 'NONE', #12210 ) ;
#23783=EDGE_CURVE ( 'NONE', #8903, #27691, #2855, .T. ) ;
#23810=DIRECTION ( 'NONE',  ( -0.000000000000000000, -1.000000000000000000, -0.000000000000000000 ) ) ;
#23816=CARTESIAN_POINT ( 'NONE',  ( -13.45329425514681532, 48.15668267613188647, -48.34811677753233283 ) ) ;
#23824=EDGE_CURVE ( 'NONE', #7501, #12057, #25422, .T. ) ;
#23869=EDGE_CURVE ( 'NONE', #20390, #21023, #20921, .T. ) ;
#23874=DIRECTION ( 'NONE',  ( -0.000000000000000000, -0.000000000000000000, 1.000000000000000000 ) ) ;
#23921=DIRECTION ( 'NONE',  ( -0.000000000000000000, -0.000000000000000000, 1.000000000000000000 ) ) ;
#23937=LINE ( 'NONE', #15033, #15945 ) ;
#23963=ORIENTED_EDGE ( 'NONE', *, *, #30716, .F. ) ;
#23969=DIRECTION ( 'NONE',  ( 0.000000000000000000, -1.000000000000000000, 0.000000000000000000 ) ) ;
#23997=ORIENTED_EDGE ( 'NONE', *, *, #9247, .F. ) ;
#23999=DIRECTION ( 'NONE',  ( -1.000000000000000000, 1.040834085586084257E-15, 0.000000000000000000 ) ) ;
#24003=EDGE_CURVE ( 'NONE', #25279, #30269, #4229, .T. ) ;
#24035=LINE ( 'NONE', #5915, #4580 ) ;
#24045=AXIS2_PLACEMENT_3D ( 'NONE', #22197, #17212, #3182 ) ;
#24056=VERTEX_POINT ( 'NONE', #14816 ) ;
#24069=AXIS2_PLACEMENT_3D ( 'NONE', #18440, #27634, #13740 ) ;
#24077=DIRECTION ( 'NONE',  ( 0.000000000000000000, 1.000000000000000000, 0.000000000000000000 ) ) ;
#24085=CARTESIAN_POINT ( 'NONE',  ( 38.00000000000000711, 90.00000000000001421, -22.50000000000002487 ) ) ;
#24104=EDGE_LOOP ( 'NONE', ( #13912, #6649, #5553, #28680 ) ) ;
#24122=ORIENTED_EDGE ( 'NONE', *, *, #15547, .F. ) ;
#24167=DIRECTION ( 'NONE',  ( -0.000000000000000000, -0.000000000000000000, -1.000000000000000000 ) ) ;
#24168=UNCERTAINTY_MEASURE_WITH_UNIT (LENGTH_MEASURE( 1.000000000000000082E-05 ), #1361, 'distance_accuracy_value', 'NONE');
#24181=ORIENTED_EDGE ( 'NONE', *, *, #27114, .T. ) ;
#24195=EDGE_CURVE ( 'NONE', #1845, #26490, #19443, .T. ) ;
#24204=EDGE_CURVE ( 'NONE', #30053, #19615, #27409, .T. ) ;
#24216=EDGE_CURVE ( 'NONE', #1741, #28813, #3589, .T. ) ;
#24225=ORIENTED_EDGE ( 'NONE', *, *, #30481, .T. ) ;
#24228=CARTESIAN_POINT ( 'NONE',  ( -37.99999999999999289, 70.00000000000000000, -75.50000000000000000 ) ) ;
#24252=VERTEX_POINT ( 'NONE', #15911 ) ;
#24273=CARTESIAN_POINT ( 'NONE',  ( 0.000000000000000000, 0.000000000000000000, -52.50000000000000000 ) ) ;
#24274=AXIS2_PLACEMENT_3D ( 'NONE', #6205, #27431, #5897 ) ;
#24288=CARTESIAN_POINT ( 'NONE',  ( -0.9972762135841950482, 50.00000000000001421, -40.00000000000002132 ) ) ;
#24324=CARTESIAN_POINT ( 'NONE',  ( 0.000000000000000000, 0.000000000000000000, -87.50000000000000000 ) ) ;
#24354=ORIENTED_EDGE ( 'NONE', *, *, #24394, .T. ) ;
#24358=CARTESIAN_POINT ( 'NONE',  ( -50.00000000000000000, -50.00000000000000000, 12.49999999999999112 ) ) ;
#24364=CARTESIAN_POINT ( 'NONE',  ( 49.99999999999998579, -70.00000000000000000, -92.50000000000000000 ) ) ;
#24374=PRODUCT_DEFINITION_SHAPE ( 'NONE', 'NONE',  #10487 ) ;
#24394=EDGE_CURVE ( 'NONE', #14635, #16844, #2476, .T. ) ;
#24404=VECTOR ( 'NONE', #12376, 1000.000000000000000 ) ;
#24411=CARTESIAN_POINT ( 'NONE',  ( -50.00000000000000000, -50.00000000000000000, 52.07879600563550326 ) ) ;
#24417=ORIENTED_EDGE ( 'NONE', *, *, #1936, .F. ) ;
#24440=CARTESIAN_POINT ( 'NONE',  ( 1.868132521858655084E-15, 50.00000000000000000, -40.00000000000000711 ) ) ;
#24512=DIRECTION ( 'NONE',  ( 0.000000000000000000, 0.000000000000000000, -1.000000000000000000 ) ) ;
#24533=EDGE_LOOP ( 'NONE', ( #30423, #14200, #16804, #20883 ) ) ;
#24544=AXIS2_PLACEMENT_3D ( 'NONE', #21439, #4603, #7247 ) ;
#24556=CARTESIAN_POINT ( 'NONE',  ( -37.99999999999999289, 70.00000000000000000, -40.50000000000000000 ) ) ;
#24593=ORIENTED_EDGE ( 'NONE', *, *, #19295, .T. ) ;
#24620=DIRECTION ( 'NONE',  ( 0.000000000000000000, 0.000000000000000000, -1.000000000000000000 ) ) ;
#24633=ORIENTED_EDGE ( 'NONE', *, *, #26762, .T. ) ;
#24649=DIRECTION ( 'NONE',  ( -0.000000000000000000, -0.000000000000000000, -1.000000000000000000 ) ) ;
#24650=FACE_OUTER_BOUND ( 'NONE', #2861, .T. ) ;
#24679=ORIENTED_EDGE ( 'NONE', *, *, #12219, .T. ) ;
#24710=CARTESIAN_POINT ( 'NONE',  ( -50.00000000000000000, 70.00000000000000000, -92.50000000000000000 ) ) ;
#24725=CARTESIAN_POINT ( 'NONE',  ( 38.00000000000000711, 70.00000000000000000, -22.50000000000003553 ) ) ;
#24731=FACE_OUTER_BOUND ( 'NONE', #18547, .T. ) ;
#24788=CARTESIAN_POINT ( 'NONE',  ( -37.99999999999999289, 209.2686044187655909, -34.49999999999999289 ) ) ;
#24843=EDGE_LOOP ( 'NONE', ( #6727, #19715 ) ) ;
#24851=CARTESIAN_POINT ( 'NONE',  ( 3.914987921652262948, 49.85603305452615075, -69.51408439781332049 ) ) ;
#24891=AXIS2_PLACEMENT_3D ( 'NONE', #14364, #23874, #5006 ) ;
#24895=CARTESIAN_POINT ( 'NONE',  ( -49.99999999999998579, 209.2686044187655909, -34.49999999999998579 ) ) ;
#24946=DIRECTION ( 'NONE',  ( 0.000000000000000000, 0.000000000000000000, -1.000000000000000000 ) ) ;
#24965=AXIS2_PLACEMENT_3D ( 'NONE', #563, #2921, #17103 ) ;
#24974=ORIENTED_EDGE ( 'NONE', *, *, #1965, .F. ) ;
#25004=CARTESIAN_POINT ( 'NONE',  ( -37.99999999999999289, 209.2686044187655909, -22.50000000000001421 ) ) ;
#25042=CARTESIAN_POINT ( 'NONE',  ( 49.99999999999998579, -50.00000000000000000, 52.07879600563550326 ) ) ;
#25049=FACE_BOUND ( 'NONE', #3814, .T. ) ;
#25055=DIRECTION ( 'NONE',  ( 0.000000000000000000, 0.000000000000000000, 1.000000000000000000 ) ) ;
#25085=CIRCLE ( 'NONE', #24069, 7.500000000000000000 ) ;
#25110=AXIS2_PLACEMENT_3D ( 'NONE', #30606, #9252, #4569 ) ;
#25121=PLANE ( 'NONE',  #1424 ) ;
#25122=VERTEX_POINT ( 'NONE', #418 ) ;
#25140=ORIENTED_EDGE ( 'NONE', *, *, #8308, .T. ) ;
#25143=UNCERTAINTY_MEASURE_WITH_UNIT (LENGTH_MEASURE( 1.000000000000000082E-05 ), #10547, 'distance_accuracy_value', 'NONE');
#25157=FACE_OUTER_BOUND ( 'NONE', #30234, .T. ) ;
#25163=EDGE_CURVE ( 'NONE', #29647, #22222, #22955, .T. ) ;
#25190=VECTOR ( 'NONE', #22601, 1000.000000000000000 ) ;
#25194=DIRECTION ( 'NONE',  ( 1.000000000000000000, 0.000000000000000000, 0.000000000000000000 ) ) ;
#25219=CIRCLE ( 'NONE', #21208, 50.00000000000000000 ) ;
#25238=CARTESIAN_POINT ( 'NONE',  ( 57.49999999999998579, -50.00000000000000000, 52.07879600563550326 ) ) ;
#25257=EDGE_LOOP ( 'NONE', ( #26385, #11203, #19156, #13507 ) ) ;
#25279=VERTEX_POINT ( 'NONE', #3538 ) ;
#25296=CARTESIAN_POINT ( 'NONE',  ( 0.000000000000000000, 0.000000000000000000, -52.50000000000000000 ) ) ;
#25297=AXIS2_PLACEMENT_3D ( 'NONE', #24411, #3053, #5544 ) ;
#25301=AXIS2_PLACEMENT_3D ( 'NONE', #26942, #10082, #5562 ) ;
#25306=DIRECTION ( 'NONE',  ( 0.000000000000000000, 0.000000000000000000, 1.000000000000000000 ) ) ;
#25312=CARTESIAN_POINT ( 'NONE',  ( 14.99996214399394567, 47.69697197601039562, -55.49547544386297204 ) ) ;
#25313=CARTESIAN_POINT ( 'NONE',  ( -50.00000000000000000, 70.00000000000000000, -75.50000000000002842 ) ) ;
#25316=DIRECTION ( 'NONE',  ( -1.000000000000000000, 0.000000000000000000, 0.000000000000000000 ) ) ;
#25341=CARTESIAN_POINT ( 'NONE',  ( -57.50000000000001421, -50.00000000000000000, 52.07879600563550326 ) ) ;
#25352=CARTESIAN_POINT ( 'NONE',  ( 0.000000000000000000, -14.99999999999997158, -55.00000000000000711 ) ) ;
#25366=CIRCLE ( 'NONE', #11926, 6.000000000000005329 ) ;
#25372=CARTESIAN_POINT ( 'NONE',  ( -50.00000000000000000, 50.00000000000000000, -92.50000000000000000 ) ) ;
#25387=ORIENTED_EDGE ( 'NONE', *, *, #30177, .F. ) ;
#25393=CARTESIAN_POINT ( 'NONE',  ( -70.00000000000000000, 70.00000000000000000, -92.50000000000000000 ) ) ;
#25422=CIRCLE ( 'NONE', #27430, 6.000000000000005329 ) ;
#25465=DIRECTION ( 'NONE',  ( 0.000000000000000000, 0.000000000000000000, 1.000000000000000000 ) ) ;
#25468=VECTOR ( 'NONE', #17673, 1000.000000000000000 ) ;
#25472=ORIENTED_EDGE ( 'NONE', *, *, #11100, .F. ) ;
#25474=CARTESIAN_POINT ( 'NONE',  ( 9.161835861599374908, 49.16032949430592680, -66.91699464352380744 ) ) ;
#25502=ORIENTED_EDGE ( 'NONE', *, *, #5764, .T. ) ;
#25532=VERTEX_POINT ( 'NONE', #8938 ) ;
#25594=ORIENTED_EDGE ( 'NONE', *, *, #26762, .F. ) ;
#25596=CARTESIAN_POINT ( 'NONE',  ( 0.000000000000000000, 0.000000000000000000, -87.50000000000000000 ) ) ;
#25610=AXIS2_PLACEMENT_3D ( 'NONE', #19363, #635, #28884 ) ;
#25622=ORIENTED_EDGE ( 'NONE', *, *, #11710, .F. ) ;
#25624=CARTESIAN_POINT ( 'NONE',  ( 9.906380082428048794, 49.01032848149721133, -43.72596795826983396 ) ) ;
#25642=FACE_OUTER_BOUND ( 'NONE', #28889, .T. ) ;
#25697=DIRECTION ( 'NONE',  ( 0.000000000000000000, 0.000000000000000000, 1.000000000000000000 ) ) ;
#25702=FACE_OUTER_BOUND ( 'NONE', #28735, .T. ) ;
#25757=DIRECTION ( 'NONE',  ( 0.000000000000000000, 0.000000000000000000, -1.000000000000000000 ) ) ;
#25771=CIRCLE ( 'NONE', #4347, 7.500000000000013323 ) ;
#25778=DIRECTION ( 'NONE',  ( 0.000000000000000000, 1.000000000000000000, 0.000000000000000000 ) ) ;
#25783=CARTESIAN_POINT ( 'NONE',  ( 49.99999999999997868, 209.2686044187655909, -34.50000000000000000 ) ) ;
#25793=CARTESIAN_POINT ( 'NONE',  ( 49.99999999999998579, 50.00000000000000000, 12.49999999999999112 ) ) ;
#25812=EDGE_LOOP ( 'NONE', ( #20181, #10779 ) ) ;
#25819=VECTOR ( 'NONE', #988, 1000.000000000000000 ) ;
#25824=FACE_OUTER_BOUND ( 'NONE', #9059, .T. ) ;
#25851=ORIENTED_EDGE ( 'NONE', *, *, #20636, .T. ) ;
#25874=EDGE_CURVE ( 'NONE', #24056, #22039, #18540, .T. ) ;
#25878=CARTESIAN_POINT ( 'NONE',  ( -12.50000000000000000, 0.000000000000000000, -87.50000000000000000 ) ) ;
#25934=ORIENTED_EDGE ( 'NONE', *, *, #27142, .F. ) ;
#25953=VERTEX_POINT ( 'NONE', #9155 ) ;
#25961=DIRECTION ( 'NONE',  ( 0.000000000000000000, 1.000000000000000000, 0.000000000000000000 ) ) ;
#26032=CARTESIAN_POINT ( 'NONE',  ( -42.49999999999998579, -50.00000000000000000, 12.49999999999999112 ) ) ;
#26047=CARTESIAN_POINT ( 'NONE',  ( 0.000000000000000000, 0.000000000000000000, -87.50000000000000000 ) ) ;
#26057=DIRECTION ( 'NONE',  ( 0.000000000000000000, 0.000000000000000000, 1.000000000000000000 ) ) ;
#26067=CARTESIAN_POINT ( 'NONE',  ( 6.674134664086328605, 49.56092362459834533, -41.53091777090556747 ) ) ;
#26113=FACE_OUTER_BOUND ( 'NONE', #29675, .T. ) ;
#26115=CARTESIAN_POINT ( 'NONE',  ( -37.99999999999999289, 209.2686044187655909, -75.50000000000000000 ) ) ;
#26122=CARTESIAN_POINT ( 'NONE',  ( -12.50000000000000000, 0.000000000000000000, -52.50000000000000000 ) ) ;
#26125=DIRECTION ( 'NONE',  ( 0.000000000000000000, 0.000000000000000000, -1.000000000000000000 ) ) ;
#26165=CARTESIAN_POINT ( 'NONE',  ( 37.99999999999999289, 70.00000000000000000, -75.50000000000001421 ) ) ;
#26166=ORIENTED_EDGE ( 'NONE', *, *, #3877, .F. ) ;
#26201=CIRCLE ( 'NONE', #16249, 32.50000000000000000 ) ;
#26247=ORIENTED_EDGE ( 'NONE', *, *, #29230, .F. ) ;
#26252=ORIENTED_EDGE ( 'NONE', *, *, #2378, .F. ) ;
#26256=VECTOR ( 'NONE', #6418, 1000.000000000000000 ) ;
#26258=CARTESIAN_POINT ( 'NONE',  ( -50.00000000000000000, 50.00000000000000000, 12.49999999999998401 ) ) ;
#26261=CARTESIAN_POINT ( 'NONE',  ( 0.000000000000000000, 0.000000000000000000, -87.50000000000000000 ) ) ;
#26268=LINE ( 'NONE', #17217, #6423 ) ;
#26289=ORIENTED_EDGE ( 'NONE', *, *, #17620, .F. ) ;
#26296=EDGE_LOOP ( 'NONE', ( #4193, #29468, #22785, #25622 ) ) ;
#26323=CARTESIAN_POINT ( 'NONE',  ( -14.49051644145457551, 47.85444022314150914, -51.09264228519022311 ) ) ;
#26334=DIRECTION ( 'NONE',  ( -0.000000000000000000, -1.000000000000000000, -0.000000000000000000 ) ) ;
#26350=EDGE_CURVE ( 'NONE', #9106, #8430, #991, .T. ) ;
#26360=CARTESIAN_POINT ( 'NONE',  ( 12.50000000000000000, 1.530808498934191521E-15, -52.50000000000000000 ) ) ;
#26385=ORIENTED_EDGE ( 'NONE', *, *, #21926, .F. ) ;
#26395=AXIS2_PLACEMENT_3D ( 'NONE', #30320, #18482, #6469 ) ;
#26397=CARTESIAN_POINT ( 'NONE',  ( 57.49999999999998579, 50.00000000000000000, -87.50000000000000000 ) ) ;
#26448=EDGE_LOOP ( 'NONE', ( #4726, #9605 ) ) ;
#26477=CARTESIAN_POINT ( 'NONE',  ( -12.73485997267505354, 48.35185223527960119, -62.94106308776442660 ) ) ;
#26490=VERTEX_POINT ( 'NONE', #25313 ) ;
#26497=LINE ( 'NONE', #15095, #16227 ) ;
#26500=DIRECTION ( 'NONE',  ( -1.000000000000000000, 0.000000000000000000, 0.000000000000000000 ) ) ;
#26510=DIRECTION ( 'NONE',  ( -1.000000000000000000, 0.000000000000000000, -0.000000000000000000 ) ) ;
#26519=VERTEX_POINT ( 'NONE', #8325 ) ;
#26545=EDGE_CURVE ( 'NONE', #18139, #11207, #12507, .T. ) ;
#26567=ORIENTED_EDGE ( 'NONE', *, *, #19528, .T. ) ;
#26609=AXIS2_PLACEMENT_3D ( 'NONE', #4258, #16426, #21086 ) ;
#26628=AXIS2_PLACEMENT_3D ( 'NONE', #24324, #24946, #7795 ) ;
#26632=CARTESIAN_POINT ( 'NONE',  ( 37.99999999999999289, 70.00000000000000000, -75.50000000000001421 ) ) ;
#26637=CARTESIAN_POINT ( 'NONE',  ( -14.61253163965172952, 47.81719550270585728, -51.57679968430688433 ) ) ;
#26646=AXIS2_PLACEMENT_3D ( 'NONE', #12375, #350, #22025 ) ;
#26689=CARTESIAN_POINT ( 'NONE',  ( -37.99999999999999289, 209.2686044187655909, -34.49999999999999289 ) ) ;
#26700=ADVANCED_FACE ( 'NONE', ( #5638 ), #29343, .T. ) ;
#26726=CARTESIAN_POINT ( 'NONE',  ( -42.49999999999998579, 50.00000000000000000, -87.50000000000000000 ) ) ;
#26742=DIRECTION ( 'NONE',  ( 1.000000000000000000, 0.000000000000000000, -1.369518533665900312E-16 ) ) ;
#26762=EDGE_CURVE ( 'NONE', #19615, #30053, #16138, .T. ) ;
#26786=DIRECTION ( 'NONE',  ( -0.000000000000000000, -1.000000000000000000, -0.000000000000000000 ) ) ;
#26800=CARTESIAN_POINT ( 'NONE',  ( -3.897762246399228303, 49.85010185758739709, -40.50684067140829114 ) ) ;
#26804=ADVANCED_FACE ( 'NONE', ( #9848 ), #7516, .T. ) ;
#26816=ORIENTED_EDGE ( 'NONE', *, *, #9015, .F. ) ;
#26822=CIRCLE ( 'NONE', #18365, 32.50000000000000000 ) ;
#26874=CIRCLE ( 'NONE', #27877, 12.50000000000000000 ) ;
#26875=PLANE ( 'NONE',  #15380 ) ;
#26881=CARTESIAN_POINT ( 'NONE',  ( 0.000000000000000000, 0.000000000000000000, 196.3477631085023631 ) ) ;
#26886=CARTESIAN_POINT ( 'NONE',  ( -37.99999999999999289, 90.00000000000001421, -22.50000000000001421 ) ) ;
#26900=ORIENTED_EDGE ( 'NONE', *, *, #11130, .T. ) ;
#26903=DIRECTION ( 'NONE',  ( 0.000000000000000000, 0.000000000000000000, -1.000000000000000000 ) ) ;
#26915=EDGE_CURVE ( 'NONE', #2444, #25279, #4059, .T. ) ;
#26942=CARTESIAN_POINT ( 'NONE',  ( -50.00000000000000000, 50.00000000000000000, -87.50000000000000000 ) ) ;
#26948=DIRECTION ( 'NONE',  ( 0.000000000000000000, 1.000000000000000000, -0.000000000000000000 ) ) ;
#26954=CARTESIAN_POINT ( 'NONE',  ( -10.26695923285440060, 48.93580713664579207, -44.05349679880919922 ) ) ;
#26980=DIRECTION ( 'NONE',  ( -0.000000000000000000, -0.000000000000000000, -1.000000000000000000 ) ) ;
#27015=VERTEX_POINT ( 'NONE', #19164 ) ;
#27017=DIRECTION ( 'NONE',  ( 0.000000000000000000, 1.000000000000000000, 0.000000000000000000 ) ) ;
#27020=EDGE_LOOP ( 'NONE', ( #4177, #4805, #14499, #15152, #13068, #29446 ) ) ;
#27029=VERTEX_POINT ( 'NONE', #28071 ) ;
#27031=ORIENTED_EDGE ( 'NONE', *, *, #10906, .F. ) ;
#27033=DIRECTION ( 'NONE',  ( 0.000000000000000000, 0.000000000000000000, 1.000000000000000000 ) ) ;
#27114=EDGE_CURVE ( 'NONE', #22222, #11207, #13879, .T. ) ;
#27142=EDGE_CURVE ( 'NONE', #17860, #1741, #28529, .T. ) ;
#27143=VERTEX_POINT ( 'NONE', #26032 ) ;
#27145=DIRECTION ( 'NONE',  ( 0.000000000000000000, -0.000000000000000000, -1.000000000000000000 ) ) ;
#27150=ORIENTED_EDGE ( 'NONE', *, *, #20636, .F. ) ;
#27176=FACE_BOUND ( 'NONE', #2192, .T. ) ;
#27202=CIRCLE ( 'NONE', #13274, 6.000000000000005329 ) ;
#27213=FACE_OUTER_BOUND ( 'NONE', #17625, .T. ) ;
#27231=CYLINDRICAL_SURFACE ( 'NONE', #10238, 7.500000000000000000 ) ;
#27242=AXIS2_PLACEMENT_3D ( 'NONE', #859, #2197, #19043 ) ;
#27251=AXIS2_PLACEMENT_3D ( 'NONE', #25596, #13739, #6101 ) ;
#27283=VECTOR ( 'NONE', #3690, 1000.000000000000000 ) ;
#27339=CIRCLE ( 'NONE', #18863, 12.50000000000000000 ) ;
#27361=DIRECTION ( 'NONE',  ( 0.000000000000000000, 0.000000000000000000, 1.000000000000000000 ) ) ;
#27371=CARTESIAN_POINT ( 'NONE',  ( -42.49999999999998579, 50.00000000000000000, 52.07879600563550326 ) ) ;
#27407=VERTEX_POINT ( 'NONE', #30662 ) ;
#27409=CIRCLE ( 'NONE', #6490, 7.500000000000013323 ) ;
#27430=AXIS2_PLACEMENT_3D ( 'NONE', #8484, #17831, #29371 ) ;
#27431=DIRECTION ( 'NONE',  ( -0.000000000000000000, -1.000000000000000000, -0.000000000000000000 ) ) ;
#27437=CARTESIAN_POINT ( 'NONE',  ( -57.50000000000001421, -50.00000000000000000, 12.49999999999999112 ) ) ;
#27463=ORIENTED_EDGE ( 'NONE', *, *, #5558, .T. ) ;
#27504=CARTESIAN_POINT ( 'NONE',  ( 14.20503062814195872, 47.93995967969133432, -50.15627268418315765 ) ) ;
#27517=ADVANCED_FACE ( 'NONE', ( #12704 ), #7715, .F. ) ;
#27536=ADVANCED_FACE ( 'NONE', ( #10193 ), #19701, .F. ) ;
#27552=DIRECTION ( 'NONE',  ( 0.000000000000000000, 0.000000000000000000, -1.000000000000000000 ) ) ;
#27555=FACE_BOUND ( 'NONE', #12921, .T. ) ;
#27558=VERTEX_POINT ( 'NONE', #7865 ) ;
#27632=AXIS2_PLACEMENT_3D ( 'NONE', #29632, #17149, #10449 ) ;
#27634=DIRECTION ( 'NONE',  ( 0.000000000000000000, 0.000000000000000000, -1.000000000000000000 ) ) ;
#27657=EDGE_CURVE ( 'NONE', #7501, #16188, #29535, .T. ) ;
#27677=DIRECTION ( 'NONE',  ( 0.000000000000000000, 0.000000000000000000, 1.000000000000000000 ) ) ;
#27680=EDGE_CURVE ( 'NONE', #22039, #24056, #5130, .T. ) ;
#27691=VERTEX_POINT ( 'NONE', #22817 ) ;
#27703=CARTESIAN_POINT ( 'NONE',  ( -37.99999999999999289, 70.00000000000000000, -81.50000000000000000 ) ) ;
#27757=ORIENTED_EDGE ( 'NONE', *, *, #17566, .F. ) ;
#27770=AXIS2_PLACEMENT_3D ( 'NONE', #20302, #29827, #17972 ) ;
#27771=ORIENTED_EDGE ( 'NONE', *, *, #3679, .T. ) ;
#27781=PLANE ( 'NONE',  #8390 ) ;
#27784=CYLINDRICAL_SURFACE ( 'NONE', #19713, 6.000000000000005329 ) ;
#27797=DIRECTION ( 'NONE',  ( 0.000000000000000000, 0.000000000000000000, 1.000000000000000000 ) ) ;
#27801=AXIS2_PLACEMENT_3D ( 'NONE', #3301, #22014, #29513 ) ;
#27816=CARTESIAN_POINT ( 'NONE',  ( 6.652725104973315595, 49.55738370017981964, -68.45305803092846020 ) ) ;
#27837=CARTESIAN_POINT ( 'NONE',  ( 37.99999999999999289, 70.00000000000000000, -75.50000000000001421 ) ) ;
#27849=DIRECTION ( 'NONE',  ( -1.000000000000000000, 0.000000000000000000, 0.000000000000000000 ) ) ;
#27877=AXIS2_PLACEMENT_3D ( 'NONE', #25296, #20748, #13746 ) ;
#27890=DIRECTION ( 'NONE',  ( 0.000000000000000000, -1.000000000000000000, 0.000000000000000000 ) ) ;
#27913=DIRECTION ( 'NONE',  ( -0.000000000000000000, -1.000000000000000000, -0.000000000000000000 ) ) ;
#28036=CARTESIAN_POINT ( 'NONE',  ( -37.99999999999999289, 90.00000000000001421, -75.50000000000000000 ) ) ;
#28046=DIRECTION ( 'NONE',  ( -1.000000000000000000, 0.000000000000000000, 0.000000000000000000 ) ) ;
#28071=CARTESIAN_POINT ( 'NONE',  ( -49.99999999999998579, 90.00000000000001421, -34.49999999999998579 ) ) ;
#28092=AXIS2_PLACEMENT_3D ( 'NONE', #25793, #16570, #11450 ) ;
#28094=EDGE_CURVE ( 'NONE', #22863, #10221, #13125, .T. ) ;
#28096=ORIENTED_EDGE ( 'NONE', *, *, #14936, .T. ) ;
#28120=DIRECTION ( 'NONE',  ( 0.000000000000000000, 0.000000000000000000, 1.000000000000000000 ) ) ;
#28131=CARTESIAN_POINT ( 'NONE',  ( 37.99999999999999289, 90.00000000000001421, -28.49999999999999645 ) ) ;
#28173=AXIS2_PLACEMENT_3D ( 'NONE', #3204, #5543, #29098 ) ;
#28175=DIRECTION ( 'NONE',  ( 0.000000000000000000, 0.000000000000000000, -1.000000000000000000 ) ) ;
#28192=EDGE_LOOP ( 'NONE', ( #15343, #4292, #12067, #17902 ) ) ;
#28201=VERTEX_POINT ( 'NONE', #7327 ) ;
#28209=ORIENTED_EDGE ( 'NONE', *, *, #28350, .F. ) ;
#28226=AXIS2_PLACEMENT_3D ( 'NONE', #7873, #26903, #3801 ) ;
#28240=AXIS2_PLACEMENT_3D ( 'NONE', #12226, #14418, #9436 ) ;
#28266=AXIS2_PLACEMENT_3D ( 'NONE', #25393, #27890, #6515 ) ;
#28272=ADVANCED_FACE ( 'NONE', ( #8642 ), #30150, .T. ) ;
#28275=LINE ( 'NONE', #13637, #13351 ) ;
#28277=EDGE_CURVE ( 'NONE', #20793, #1845, #21075, .T. ) ;
#28348=ORIENTED_EDGE ( 'NONE', *, *, #431, .T. ) ;
#28350=EDGE_CURVE ( 'NONE', #8430, #23138, #28275, .T. ) ;
#28391=FACE_BOUND ( 'NONE', #1045, .T. ) ;
#28394=ORIENTED_EDGE ( 'NONE', *, *, #15667, .F. ) ;
#28398=CARTESIAN_POINT ( 'NONE',  ( 37.99999999999999289, 209.2686044187655909, -69.50000000000000000 ) ) ;
#28415=CARTESIAN_POINT ( 'NONE',  ( 7.532524345205997562, 49.43623389526102585, -41.99159057664593320 ) ) ;
#28429=LINE ( 'NONE', #9094, #30488 ) ;
#28461=EDGE_CURVE ( 'NONE', #18599, #15417, #3888, .T. ) ;
#28482=VERTEX_POINT ( 'NONE', #2642 ) ;
#28489=ADVANCED_FACE ( 'NONE', ( #16525, #28391 ), #2327, .F. ) ;
#28514=DIRECTION ( 'NONE',  ( 0.000000000000000000, 0.000000000000000000, 1.000000000000000000 ) ) ;
#28529=LINE ( 'NONE', #28684, #16568 ) ;
#28542=ORIENTED_EDGE ( 'NONE', *, *, #5062, .F. ) ;
#28556=ORIENTED_EDGE ( 'NONE', *, *, #24195, .T. ) ;
#28560=CARTESIAN_POINT ( 'NONE',  ( -37.99999999999999289, 90.00000000000001421, -28.49999999999998934 ) ) ;
#28665=CARTESIAN_POINT ( 'NONE',  ( 69.99999999999998579, 50.00000000000000000, -92.50000000000000000 ) ) ;
#28666=CARTESIAN_POINT ( 'NONE',  ( -10.94934520787159826, 48.78767624520369139, -65.26408404810210584 ) ) ;
#28680=ORIENTED_EDGE ( 'NONE', *, *, #27657, .F. ) ;
#28684=CARTESIAN_POINT ( 'NONE',  ( 69.99999999999998579, -70.00000000000000000, 12.49999999999999112 ) ) ;
#28693=LINE ( 'NONE', #30418, #21702 ) ;
#28735=EDGE_LOOP ( 'NONE', ( #22846, #21205, #28556, #27757 ) ) ;
#28752=ORIENTED_EDGE ( 'NONE', *, *, #15458, .F. ) ;
#28769=PLANE ( 'NONE',  #937 ) ;
#28809=DIRECTION ( 'NONE',  ( 0.000000000000000000, 0.000000000000000000, 1.000000000000000000 ) ) ;
#28813=VERTEX_POINT ( 'NONE', #7442 ) ;
#28861=DIRECTION ( 'NONE',  ( -0.000000000000000000, -0.000000000000000000, 1.000000000000000000 ) ) ;
#28884=DIRECTION ( 'NONE',  ( 0.000000000000000000, 0.000000000000000000, -1.000000000000000000 ) ) ;
#28889=EDGE_LOOP ( 'NONE', ( #17539, #13453, #29555, #12391 ) ) ;
#28914=EDGE_LOOP ( 'NONE', ( #14047, #3550 ) ) ;
#28948=CYLINDRICAL_SURFACE ( 'NONE', #28173, 7.500000000000000000 ) ;
#28960=DIRECTION ( 'NONE',  ( -0.000000000000000000, -1.000000000000000000, -0.000000000000000000 ) ) ;
#28963=DIRECTION ( 'NONE',  ( -1.000000000000000000, 0.000000000000000000, 0.000000000000000000 ) ) ;
#28973=CARTESIAN_POINT ( 'NONE',  ( -11.91668235487185257, 48.56246597984248581, -45.83682539780265586 ) ) ;
#28981=CARTESIAN_POINT ( 'NONE',  ( 37.99999999999999289, 209.2686044187655909, -81.50000000000001421 ) ) ;
#29009=EDGE_LOOP ( 'NONE', ( #9075, #10849, #10037, #26166 ) ) ;
#29054=ORIENTED_EDGE ( 'NONE', *, *, #21985, .F. ) ;
#29068=CARTESIAN_POINT ( 'NONE',  ( 42.49999999999998579, 50.00000000000000000, 12.49999999999999112 ) ) ;
#29098=DIRECTION ( 'NONE',  ( -1.000000000000000000, 0.000000000000000000, 0.000000000000000000 ) ) ;
#29112=CARTESIAN_POINT ( 'NONE',  ( 49.99999999999998579, 70.00000000000000000, -92.50000000000000000 ) ) ;
#29116=CIRCLE ( 'NONE', #27632, 7.500000000000000000 ) ;
#29121=CARTESIAN_POINT ( 'NONE',  ( 0.000000000000000000, 90.00000000000001421, -40.00000000000000711 ) ) ;
#29123=ORIENTED_EDGE ( 'NONE', *, *, #431, .F. ) ;
#29138=FACE_OUTER_BOUND ( 'NONE', #29009, .T. ) ;
#29150=EDGE_CURVE ( 'NONE', #22434, #11709, #26822, .T. ) ;
#29160=PLANE ( 'NONE',  #11677 ) ;
#29161=CARTESIAN_POINT ( 'NONE',  ( -70.00000000000000000, 50.00000000000000000, 12.49999999999999112 ) ) ;
#29175=EDGE_CURVE ( 'NONE', #3976, #11851, #7089, .T. ) ;
#29187=CARTESIAN_POINT ( 'NONE',  ( 37.99999999999999289, 90.00000000000001421, -75.50000000000001421 ) ) ;
#29214=ORIENTED_EDGE ( 'NONE', *, *, #16258, .F. ) ;
#29230=EDGE_CURVE ( 'NONE', #26490, #24252, #10045, .T. ) ;
#29243=CARTESIAN_POINT ( 'NONE',  ( -50.00000000000000000, -50.00000000000000000, -92.50000000000000000 ) ) ;
#29249=VECTOR ( 'NONE', #10226, 1000.000000000000000 ) ;
#29266=ORIENTED_EDGE ( 'NONE', *, *, #20, .F. ) ;
#29274=DIRECTION ( 'NONE',  ( 0.000000000000000000, 0.4961389383568337030, -0.8682431421244592995 ) ) ;
#29285=CARTESIAN_POINT ( 'NONE',  ( -4.843246358613172653, 49.76713946421946133, -40.79481846074538254 ) ) ;
#29330=AXIS2_PLACEMENT_3D ( 'NONE', #9895, #9732, #3033 ) ;
#29343=CYLINDRICAL_SURFACE ( 'NONE', #5182, 32.50000000000000000 ) ;
#29365=FACE_BOUND ( 'NONE', #13447, .T. ) ;
#29368=ORIENTED_EDGE ( 'NONE', *, *, #26350, .F. ) ;
#29371=DIRECTION ( 'NONE',  ( 0.000000000000000000, 0.000000000000000000, 1.000000000000000000 ) ) ;
#29377=DIRECTION ( 'NONE',  ( -0.000000000000000000, -0.000000000000000000, -1.000000000000000000 ) ) ;
#29387=DIRECTION ( 'NONE',  ( -1.369518533665900065E-16, 0.000000000000000000, -1.000000000000000000 ) ) ;
#29422=CARTESIAN_POINT ( 'NONE',  ( 49.99999999999998579, 70.00000000000000000, -92.50000000000000000 ) ) ;
#29430=CARTESIAN_POINT ( 'NONE',  ( -37.99999999999999289, 70.00000000000000000, -87.50000000000000000 ) ) ;
#29431=DIRECTION ( 'NONE',  ( 0.000000000000000000, -0.8682431421244592995, -0.4961389383568337030 ) ) ;
#29433=CARTESIAN_POINT ( 'NONE',  ( 0.000000000000000000, 90.00000000000001421, -55.00000000000000711 ) ) ;
#29446=ORIENTED_EDGE ( 'NONE', *, *, #14922, .F. ) ;
#29468=ORIENTED_EDGE ( 'NONE', *, *, #29627, .T. ) ;
#29472=DIRECTION ( 'NONE',  ( 1.000000000000000000, 0.000000000000000000, 0.000000000000000000 ) ) ;
#29513=DIRECTION ( 'NONE',  ( 0.000000000000000000, 0.000000000000000000, 1.000000000000000000 ) ) ;
#29524=VECTOR ( 'NONE', #8265, 1000.000000000000000 ) ;
#29526=ORIENTED_EDGE ( 'NONE', *, *, #30153, .T. ) ;
#29535=LINE ( 'NONE', #8172, #14600 ) ;
#29555=ORIENTED_EDGE ( 'NONE', *, *, #12419, .F. ) ;
#29591=CARTESIAN_POINT ( 'NONE',  ( -1.967529318552797335, 49.96369992636662971, -69.87862445765860286 ) ) ;
#29613=FACE_OUTER_BOUND ( 'NONE', #8237, .T. ) ;
#29616=CARTESIAN_POINT ( 'NONE',  ( -37.99999999999999289, 90.00000000000001421, -87.50000000000000000 ) ) ;
#29627=EDGE_CURVE ( 'NONE', #22863, #18599, #26268, .T. ) ;
#29632=CARTESIAN_POINT ( 'NONE',  ( 49.99999999999998579, 50.00000000000000000, -87.50000000000000000 ) ) ;
#29638=DIRECTION ( 'NONE',  ( -0.000000000000000000, -0.000000000000000000, -1.000000000000000000 ) ) ;
#29647=VERTEX_POINT ( 'NONE', #2877 ) ;
#29675=EDGE_LOOP ( 'NONE', ( #17514, #12613, #444, #5894 ) ) ;
#29681=CARTESIAN_POINT ( 'NONE',  ( 1.962661427741273945, 49.96387296952570267, -69.87920469685937519 ) ) ;
#29706=DIRECTION ( 'NONE',  ( 0.000000000000000000, -1.000000000000000000, 0.000000000000000000 ) ) ;
#29719=DIRECTION ( 'NONE',  ( -0.000000000000000000, -0.000000000000000000, -1.000000000000000000 ) ) ;
#29726=CARTESIAN_POINT ( 'NONE',  ( -49.99999999999998579, 90.00000000000001421, -75.50000000000002842 ) ) ;
#29752=ADVANCED_FACE ( 'NONE', ( #2573 ), #9588, .F. ) ;
#29764=ADVANCED_FACE ( 'NONE', ( #26113 ), #28769, .F. ) ;
#29767=CARTESIAN_POINT ( 'NONE',  ( 0.000000000000000000, 0.000000000000000000, -87.50000000000000000 ) ) ;
#29783=ORIENTED_EDGE ( 'NONE', *, *, #11100, .T. ) ;
#29793=EDGE_CURVE ( 'NONE', #2233, #16863, #21263, .T. ) ;
#29816=VECTOR ( 'NONE', #20505, 1000.000000000000000 ) ;
#29821=DIRECTION ( 'NONE',  ( -0.000000000000000000, -1.000000000000000000, -0.000000000000000000 ) ) ;
#29827=DIRECTION ( 'NONE',  ( 0.000000000000000000, 0.000000000000000000, 1.000000000000000000 ) ) ;
#29851=CARTESIAN_POINT ( 'NONE',  ( 13.47544704454163522, 48.15148052472740403, -48.33895490383400073 ) ) ;
#29883=DIRECTION ( 'NONE',  ( 0.000000000000000000, 0.000000000000000000, -1.000000000000000000 ) ) ;
#29893=CARTESIAN_POINT ( 'NONE',  ( -50.00000000000000000, 50.00000000000000000, 52.07879600563550326 ) ) ;
#29896=CARTESIAN_POINT ( 'NONE',  ( 35.00000000000000000, 70.00000000000000000, 12.49999999999999112 ) ) ;
#29908=CARTESIAN_POINT ( 'NONE',  ( -2.462452140056639038, 49.94168384355573664, -69.80474203353597318 ) ) ;
#29960=ORIENTED_EDGE ( 'NONE', *, *, #8434, .F. ) ;
#29980=FACE_BOUND ( 'NONE', #5232, .T. ) ;
#30038=CARTESIAN_POINT ( 'NONE',  ( 35.00000000000000000, 70.00000000000000000, 12.49999999999999112 ) ) ;
#30053=VERTEX_POINT ( 'NONE', #547 ) ;
#30057=DIRECTION ( 'NONE',  ( 0.000000000000000000, 0.000000000000000000, 1.000000000000000000 ) ) ;
#30060=ORIENTED_EDGE ( 'NONE', *, *, #7815, .F. ) ;
#30089=LINE ( 'NONE', #11379, #715 ) ;
#30111=ADVANCED_FACE ( 'NONE', ( #19899 ), #2908, .F. ) ;
#30148=ORIENTED_EDGE ( 'NONE', *, *, #11495, .F. ) ;
#30150=PLANE ( 'NONE',  #4873 ) ;
#30153=EDGE_CURVE ( 'NONE', #8558, #19615, #1494, .T. ) ;
#30158=CARTESIAN_POINT ( 'NONE',  ( -70.00000000000000000, 50.00000000000000000, -92.50000000000000000 ) ) ;
#30165=EDGE_LOOP ( 'NONE', ( #23175, #1241 ) ) ;
#30166=CARTESIAN_POINT ( 'NONE',  ( 0.000000000000000000, 0.000000000000000000, -52.50000000000000000 ) ) ;
#30171=DIRECTION ( 'NONE',  ( 0.000000000000000000, 1.000000000000000000, 6.938893903907227392E-16 ) ) ;
#30172=( GEOMETRIC_REPRESENTATION_CONTEXT ( 3 ) GLOBAL_UNCERTAINTY_ASSIGNED_CONTEXT ( ( #25143 ) ) GLOBAL_UNIT_ASSIGNED_CONTEXT ( ( #10547, #22078, #3214 ) ) REPRESENTATION_CONTEXT ( 'NONE', 'WORKASPACE' ) );
#30177=EDGE_CURVE ( 'NONE', #13645, #23441, #13505, .T. ) ;
#30178=CARTESIAN_POINT ( 'NONE',  ( -49.99999999999998579, 90.00000000000001421, -75.50000000000002842 ) ) ;
#30193=VECTOR ( 'NONE', #14285, 1000.000000000000000 ) ;
#30231=AXIS2_PLACEMENT_3D ( 'NONE', #8610, #18439, #9061 ) ;
#30234=EDGE_LOOP ( 'NONE', ( #28542, #4671 ) ) ;
#30239=LINE ( 'NONE', #11954, #18566 ) ;
#30263=DIRECTION ( 'NONE',  ( 0.000000000000000000, 0.000000000000000000, -1.000000000000000000 ) ) ;
#30269=VERTEX_POINT ( 'NONE', #20651 ) ;
#30278=VECTOR ( 'NONE', #2650, 1000.000000000000000 ) ;
#30293=VECTOR ( 'NONE', #11607, 1000.000000000000000 ) ;
#30294=CARTESIAN_POINT ( 'NONE',  ( 12.19428753565139090, 48.49100318506136631, -63.74847735431697515 ) ) ;
#30313=CARTESIAN_POINT ( 'NONE',  ( 49.99999999999998579, 70.00000000000000000, -34.50000000000000000 ) ) ;
#30320=CARTESIAN_POINT ( 'NONE',  ( 49.99999999999998579, -50.00000000000000000, -92.50000000000000000 ) ) ;
#30360=CARTESIAN_POINT ( 'NONE',  ( -37.99999999999999289, 70.00000000000000000, -28.49999999999998934 ) ) ;
#30363=EDGE_CURVE ( 'NONE', #27143, #8558, #2873, .T. ) ;
#30373=EDGE_CURVE ( 'NONE', #6658, #2444, #20310, .T. ) ;
#30392=ORIENTED_EDGE ( 'NONE', *, *, #1570, .T. ) ;
#30404=ORIENTED_EDGE ( 'NONE', *, *, #29793, .T. ) ;
#30418=CARTESIAN_POINT ( 'NONE',  ( 37.99999999999999289, 209.2686044187655909, -40.50000000000000711 ) ) ;
#30423=ORIENTED_EDGE ( 'NONE', *, *, #23477, .F. ) ;
#30424=PLANE ( 'NONE',  #30231 ) ;
#30443=CARTESIAN_POINT ( 'NONE',  ( 3.424950581212853784, 49.88489954546552951, -40.38796021397682523 ) ) ;
#30449=CARTESIAN_POINT ( 'NONE',  ( -35.00000000000000000, 0.000000000000000000, 0.000000000000000000 ) ) ;
#30467=VECTOR ( 'NONE', #9869, 1000.000000000000000 ) ;
#30470=CARTESIAN_POINT ( 'NONE',  ( 0.000000000000000000, 0.000000000000000000, 12.49999999999998401 ) ) ;
#30479=DIRECTION ( 'NONE',  ( 1.000000000000000000, 0.000000000000000000, 0.000000000000000000 ) ) ;
#30481=EDGE_CURVE ( 'NONE', #2772, #11709, #21048, .T. ) ;
#30488=VECTOR ( 'NONE', #1767, 1000.000000000000000 ) ;
#30503=EDGE_CURVE ( 'NONE', #28482, #9112, #18887, .T. ) ;
#30507=VECTOR ( 'NONE', #7537, 1000.000000000000000 ) ;
#30519=CARTESIAN_POINT ( 'NONE',  ( 1.837104849652355830E-15, 50.00000000000000000, -70.00000000000000000 ) ) ;
#30555=CARTESIAN_POINT ( 'NONE',  ( -57.50000000000001421, 50.00000000000000000, 52.07879600563550326 ) ) ;
#30606=CARTESIAN_POINT ( 'NONE',  ( -50.00000000000000000, -50.00000000000000000, 12.49999999999999112 ) ) ;
#30621=DIRECTION ( 'NONE',  ( 0.000000000000000000, 1.000000000000000000, 0.000000000000000000 ) ) ;
#30632=DIRECTION ( 'NONE',  ( -0.000000000000000000, -1.000000000000000000, -0.000000000000000000 ) ) ;
#30657=DIRECTION ( 'NONE',  ( -1.000000000000000000, 0.000000000000000000, 0.000000000000000000 ) ) ;
#30662=CARTESIAN_POINT ( 'NONE',  ( 1.836970198721029589E-15, 90.00000000000001421, -70.00000000000000000 ) ) ;
#30665=MECHANICAL_DESIGN_GEOMETRIC_PRESENTATION_REPRESENTATION('',(#17719),#30172);
#30667=CARTESIAN_POINT ( 'NONE',  ( -50.00000000000000000, 50.00000000000000000, 52.07879600563550326 ) ) ;
#30670=ORIENTED_EDGE ( 'NONE', *, *, #7813, .F. ) ;
#30685=ORIENTED_EDGE ( 'NONE', *, *, #22919, .T. ) ;
#30716=EDGE_CURVE ( 'NONE', #8853, #10182, #19344, .T. ) ;
#30742=CIRCLE ( 'NONE', #12326, 20.00000000000000355 ) ;
#30757=ORIENTED_EDGE ( 'NONE', *, *, #18588, .F. ) ;
#30763=EDGE_CURVE ( 'NONE', #9112, #16844, #9370, .T. ) ;
#30786=AXIS2_PLACEMENT_3D ( 'NONE', #9815, #26980, #26500 ) ;
#30788=DIRECTION ( 'NONE',  ( 0.000000000000000000, 0.000000000000000000, 1.000000000000000000 ) ) ;
#30792=ORIENTED_EDGE ( 'NONE', *, *, #8786, .T. ) ;
#30873=COLOUR_RGB('Dark Blue',0.08,0.2,0.34);
#30874=FILL_AREA_STYLE_COLOUR('',#30873);
#30875=FILL_AREA_STYLE('',(#30874));
#30876=SURFACE_STYLE_FILL_AREA(#30875);
#30877=SURFACE_SIDE_STYLE('',(#30876));
#30878=SURFACE_STYLE_USAGE(.BOTH.,#30877);
#30879=PRESENTATION_STYLE_ASSIGNMENT((#30878));
ENDSEC;
END-ISO-10303-21;
